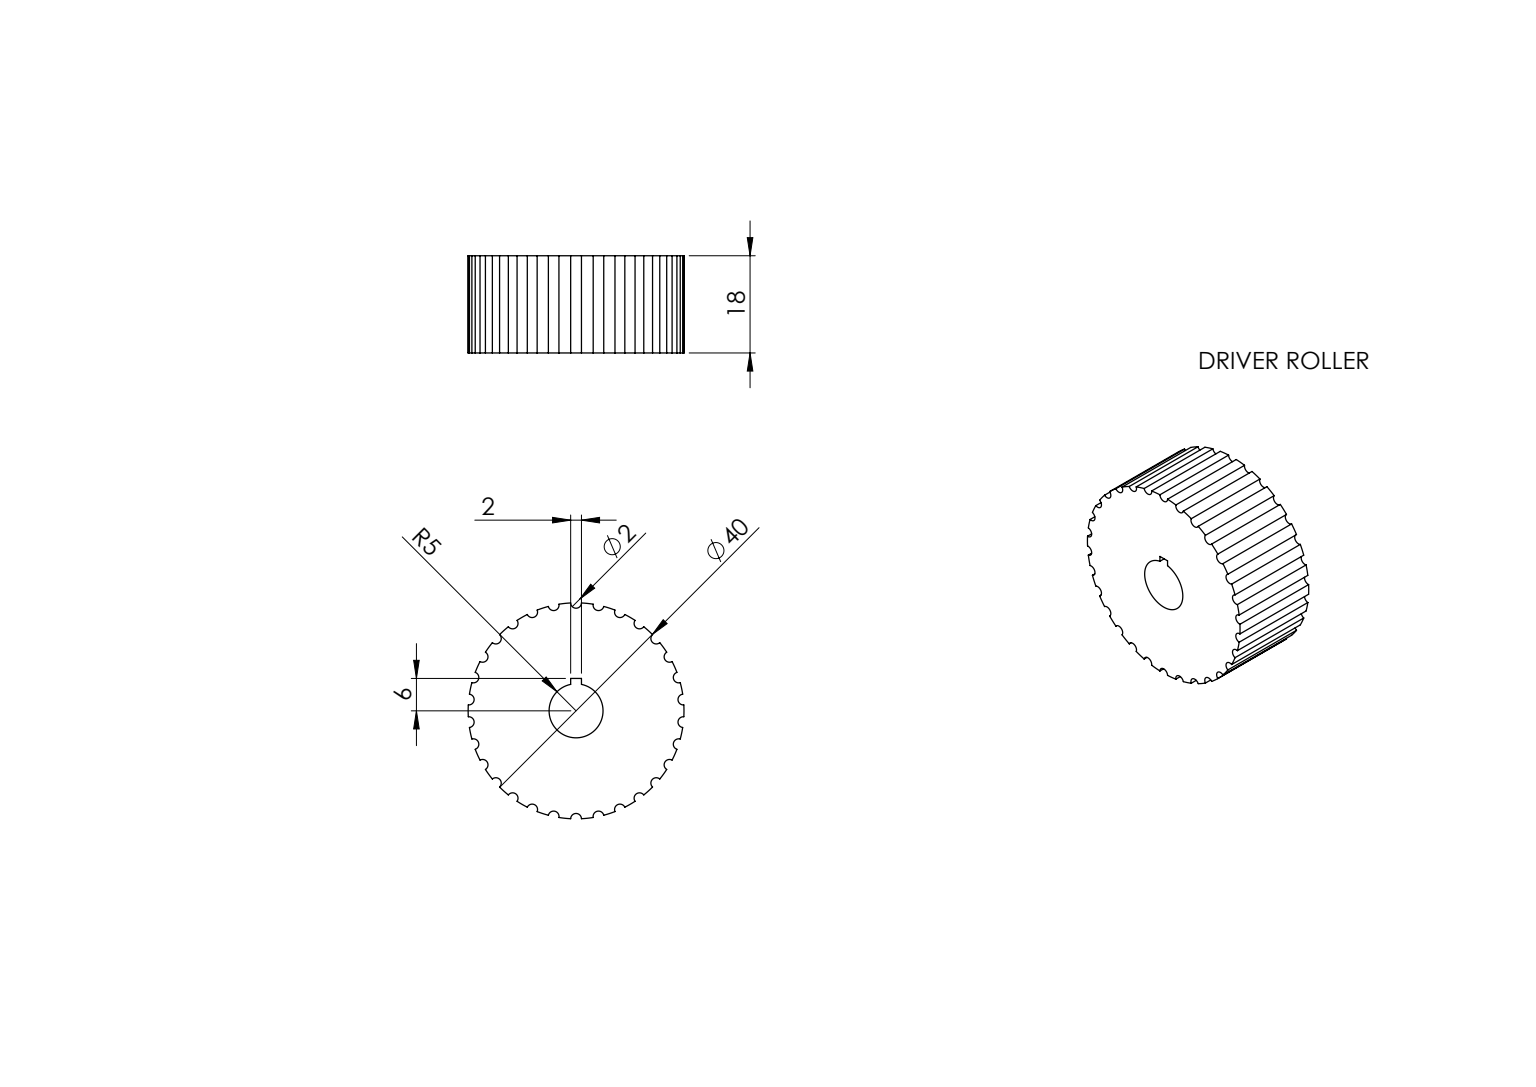
ISO-10303-21;
HEADER;
FILE_DESCRIPTION (('STEP AP214'),
    '1' );
FILE_NAME ('driver roller.step',
    '2026-10-31T03:44:21',
    ( '' ),
    ( '' ),
    'SwSTEP 2.0',
    'SolidWorks 2026',
    '' );
FILE_SCHEMA (( 'AUTOMOTIVE_DESIGN' ));
ENDSEC;

DATA;
#2=ORIENTED_EDGE ( 'NONE', *, *, #6633, .F. ) ;
#14=DIRECTION ( 'NONE',  ( -4.082155997157844188E-16, 1.000000000000000000, 0.000000000000000000 ) ) ;
#47=ORIENTED_EDGE ( 'NONE', *, *, #5852, .F. ) ;
#49=DIRECTION ( 'NONE',  ( -0.000000000000000000, -0.000000000000000000, -1.000000000000000000 ) ) ;
#61=FACE_OUTER_BOUND ( 'NONE', #9370, .T. ) ;
#94=EDGE_LOOP ( 'NONE', ( #13981, #857, #13951, #13577 ) ) ;
#95=DIRECTION ( 'NONE',  ( -1.000000000000000000, 0.000000000000000000, 0.000000000000000000 ) ) ;
#96=ORIENTED_EDGE ( 'NONE', *, *, #2338, .F. ) ;
#114=ORIENTED_EDGE ( 'NONE', *, *, #10804, .F. ) ;
#116=EDGE_CURVE ( 'NONE', #14983, #12413, #19360, .T. ) ;
#117=DIRECTION ( 'NONE',  ( 0.000000000000000000, 0.000000000000000000, 1.000000000000000000 ) ) ;
#121=CARTESIAN_POINT ( 'NONE',  ( -0.9999999999999995559, -15.10102051443364246, 9.000000000000000000 ) ) ;
#129=ORIENTED_EDGE ( 'NONE', *, *, #17684, .F. ) ;
#132=AXIS2_PLACEMENT_3D ( 'NONE', #16115, #16207, #5718 ) ;
#142=DIRECTION ( 'NONE',  ( -0.9781476007338065770, 0.2079116908177552348, 0.000000000000000000 ) ) ;
#145=CIRCLE ( 'NONE', #8274, 20.00000000000000000 ) ;
#152=CARTESIAN_POINT ( 'NONE',  ( 11.75570504584926468, -3.819660112500910198, 9.000000000000000000 ) ) ;
#159=DIRECTION ( 'NONE',  ( 1.000000000000000000, 0.000000000000000000, 0.000000000000000000 ) ) ;
#176=EDGE_CURVE ( 'NONE', #16215, #3087, #11160, .T. ) ;
#177=DIRECTION ( 'NONE',  ( 0.000000000000000000, 0.000000000000000000, 1.000000000000000000 ) ) ;
#179=ORIENTED_EDGE ( 'NONE', *, *, #18456, .F. ) ;
#183=CIRCLE ( 'NONE', #15507, 5.000000000000000888 ) ;
#193=CARTESIAN_POINT ( 'NONE',  ( -3.158233816355059620, -39.56295201467614220, -9.000000000000000000 ) ) ;
#198=CIRCLE ( 'NONE', #9874, 1.000000000000000000 ) ;
#199=CARTESIAN_POINT ( 'NONE',  ( -19.30627432446647163, -14.77814480204146363, 9.000000000000000000 ) ) ;
#209=ORIENTED_EDGE ( 'NONE', *, *, #14535, .T. ) ;
#214=DIRECTION ( 'NONE',  ( -0.000000000000000000, 0.000000000000000000, 1.000000000000000000 ) ) ;
#225=ORIENTED_EDGE ( 'NONE', *, *, #17454, .F. ) ;
#233=DIRECTION ( 'NONE',  ( -0.3090169943749528914, 0.9510565162951518658, 0.000000000000000000 ) ) ;
#250=DIRECTION ( 'NONE',  ( 0.000000000000000000, 0.000000000000000000, 1.000000000000000000 ) ) ;
#256=ORIENTED_EDGE ( 'NONE', *, *, #7357, .T. ) ;
#258=VERTEX_POINT ( 'NONE', #12266 ) ;
#274=DIRECTION ( 'NONE',  ( -0.6691306063588506881, -0.7431448254774009055, 0.000000000000000000 ) ) ;
#277=DIRECTION ( 'NONE',  ( 1.000000000000000000, 0.000000000000000000, 0.000000000000000000 ) ) ;
#279=ORIENTED_EDGE ( 'NONE', *, *, #12618, .T. ) ;
#281=EDGE_CURVE ( 'NONE', #8618, #8760, #1727, .T. ) ;
#300=FACE_OUTER_BOUND ( 'NONE', #17953, .T. ) ;
#309=DIRECTION ( 'NONE',  ( -0.000000000000000000, -0.000000000000000000, -1.000000000000000000 ) ) ;
#310=ORIENTED_EDGE ( 'NONE', *, *, #4548, .T. ) ;
#313=CIRCLE ( 'NONE', #4397, 1.000000000000000444 ) ;
#317=DIRECTION ( 'NONE',  ( 0.000000000000000000, 0.000000000000000000, 1.000000000000000000 ) ) ;
#327=CARTESIAN_POINT ( 'NONE',  ( 0.000000000000000000, 0.000000000000000000, -9.000000000000000000 ) ) ;
#329=ORIENTED_EDGE ( 'NONE', *, *, #6092, .T. ) ;
#337=VERTEX_POINT ( 'NONE', #4121 ) ;
#348=DIRECTION ( 'NONE',  ( -0.000000000000000000, -0.000000000000000000, -1.000000000000000000 ) ) ;
#354=ORIENTED_EDGE ( 'NONE', *, *, #1026, .F. ) ;
#368=FACE_OUTER_BOUND ( 'NONE', #2307, .T. ) ;
#376=DIRECTION ( 'NONE',  ( -0.000000000000000000, -0.000000000000000000, 1.000000000000000000 ) ) ;
#382=AXIS2_PLACEMENT_3D ( 'NONE', #14726, #11588, #19073 ) ;
#383=DIRECTION ( 'NONE',  ( 0.000000000000000000, 0.000000000000000000, 1.000000000000000000 ) ) ;
#388=ORIENTED_EDGE ( 'NONE', *, *, #14666, .F. ) ;
#392=DIRECTION ( 'NONE',  ( 0.000000000000000000, 0.000000000000000000, -1.000000000000000000 ) ) ;
#399=( LENGTH_UNIT ( ) NAMED_UNIT ( * ) SI_UNIT ( .MILLI., .METRE. ) );
#403=DIRECTION ( 'NONE',  ( 0.000000000000000000, 0.000000000000000000, -1.000000000000000000 ) ) ;
#408=DIRECTION ( 'NONE',  ( 0.000000000000000000, 0.000000000000000000, 1.000000000000000000 ) ) ;
#428=ORIENTED_EDGE ( 'NONE', *, *, #9768, .T. ) ;
#437=DIRECTION ( 'NONE',  ( 0.000000000000000000, 0.000000000000000000, 1.000000000000000000 ) ) ;
#438=CIRCLE ( 'NONE', #9207, 1.000000000000000222 ) ;
#439=VERTEX_POINT ( 'NONE', #4586 ) ;
#462=DIRECTION ( 'NONE',  ( 0.000000000000000000, 0.000000000000000000, 1.000000000000000000 ) ) ;
#469=FACE_OUTER_BOUND ( 'NONE', #1033, .T. ) ;
#494=CIRCLE ( 'NONE', #15524, 1.000000000000000666 ) ;
#508=VERTEX_POINT ( 'NONE', #6242 ) ;
#513=DIRECTION ( 'NONE',  ( 0.9781476007338055778, 0.2079116908177597867, 0.000000000000000000 ) ) ;
#520=CARTESIAN_POINT ( 'NONE',  ( -19.97007065299861850, -18.90625500492885180, -9.000000000000000000 ) ) ;
#526=DIRECTION ( 'NONE',  ( -0.000000000000000000, -0.000000000000000000, 1.000000000000000000 ) ) ;
#538=CARTESIAN_POINT ( 'NONE',  ( -14.17539641854921229, -5.891203581560112923, 9.000000000000000000 ) ) ;
#542=CARTESIAN_POINT ( 'NONE',  ( -0.9996874511566050669, -39.97499999999999432, 9.000000000000000000 ) ) ;
#543=ORIENTED_EDGE ( 'NONE', *, *, #13837, .F. ) ;
#550=DIRECTION ( 'NONE',  ( -0.000000000000000000, 0.000000000000000000, -1.000000000000000000 ) ) ;
#555=CARTESIAN_POINT ( 'NONE',  ( -1.000000000000000000, -14.00000000000000000, 8.999999999999998224 ) ) ;
#564=ORIENTED_EDGE ( 'NONE', *, *, #16830, .T. ) ;
#567=CARTESIAN_POINT ( 'NONE',  ( 17.79870116617236420, -10.87825472854593301, 9.000000000000000000 ) ) ;
#571=CARTESIAN_POINT ( 'NONE',  ( 18.68843350152500093, -27.12337372732038432, 0.000000000000000000 ) ) ;
#575=EDGE_CURVE ( 'NONE', #17511, #6795, #14148, .T. ) ;
#583=( NAMED_UNIT ( * ) SI_UNIT ( $, .STERADIAN. ) SOLID_ANGLE_UNIT ( ) );
#585=VERTEX_POINT ( 'NONE', #10450 ) ;
#595=LINE ( 'NONE', #15210, #9936 ) ;
#597=CARTESIAN_POINT ( 'NONE',  ( -10.93224627749309796, -3.252283996668733135, 0.000000000000000000 ) ) ;
#620=CARTESIAN_POINT ( 'NONE',  ( -11.75570504584948139, -3.819660112501066518, -9.000000000000000000 ) ) ;
#625=CIRCLE ( 'NONE', #12841, 20.00000000000000000 ) ;
#630=ORIENTED_EDGE ( 'NONE', *, *, #16372, .F. ) ;
#632=CIRCLE ( 'NONE', #5645, 1.000000000000000000 ) ;
#634=FACE_OUTER_BOUND ( 'NONE', #11741, .T. ) ;
#637=EDGE_LOOP ( 'NONE', ( #3972, #2, #1409, #7912 ) ) ;
#660=VERTEX_POINT ( 'NONE', #9650 ) ;
#661=CARTESIAN_POINT ( 'NONE',  ( -9.037824375505556063, -2.158539001597498341, 9.000000000000000000 ) ) ;
#666=VERTEX_POINT ( 'NONE', #11028 ) ;
#667=ORIENTED_EDGE ( 'NONE', *, *, #12974, .T. ) ;
#668=DIRECTION ( 'NONE',  ( -0.6691306063588624564, 0.7431448254773903583, 0.000000000000000000 ) ) ;
#673=ORIENTED_EDGE ( 'NONE', *, *, #4548, .F. ) ;
#677=CARTESIAN_POINT ( 'NONE',  ( -18.89043790736547379, -17.90943073464699609, -9.000000000000000000 ) ) ;
#681=VECTOR ( 'NONE', #14209, 1000.000000000000000 ) ;
#686=FACE_OUTER_BOUND ( 'NONE', #12366, .T. ) ;
#695=DIRECTION ( 'NONE',  ( 1.000000000000000000, 0.000000000000000000, 0.000000000000000000 ) ) ;
#716=CARTESIAN_POINT ( 'NONE',  ( -4.158233816355060064, -39.56295201467614220, 9.000000000000000000 ) ) ;
#721=CARTESIAN_POINT ( 'NONE',  ( 17.32050807568887052, -29.99999999999984013, 9.000000000000000000 ) ) ;
#727=ORIENTED_EDGE ( 'NONE', *, *, #14442, .F. ) ;
#747=CARTESIAN_POINT ( 'NONE',  ( 2.449293598294706513E-15, -20.00000000000000000, -9.000000000000000000 ) ) ;
#753=CIRCLE ( 'NONE', #14189, 20.00000000000000000 ) ;
#756=ORIENTED_EDGE ( 'NONE', *, *, #9160, .F. ) ;
#761=CARTESIAN_POINT ( 'NONE',  ( 19.76107906696387317, -16.91783288752825243, -9.000000000000000000 ) ) ;
#765=CARTESIAN_POINT ( 'NONE',  ( -4.999999999999998224, -20.00000000000000000, -8.999999999999998224 ) ) ;
#776=DIRECTION ( 'NONE',  ( -1.000000000000000000, 0.000000000000000000, 0.000000000000000000 ) ) ;
#777=SURFACE_STYLE_FILL_AREA ( #6555 ) ;
#783=EDGE_CURVE ( 'NONE', #14027, #16215, #3977, .T. ) ;
#791=CARTESIAN_POINT ( 'NONE',  ( -11.75570504584948139, -3.819660112501066518, -9.000000000000000000 ) ) ;
#811=CARTESIAN_POINT ( 'NONE',  ( 3.175194142251959395, -0.2536549670829222891, 0.000000000000000000 ) ) ;
#826=EDGE_LOOP ( 'NONE', ( #10240, #13120, #5556, #14929, #17534, #17311, #15195, #957, #13396, #3693, #849, #8118, #17435, #10866, #18404, #3444, #17944, #1819, #10052, #1799, #14812, #13494, #6030, #667, #4210, #4378, #19128, #14482, #9173, #14661, #18119, #5853, #10615, #17650, #8610, #6461, #354, #8873, #329, #14105, #1118, #11724, #12303, #13901, #12807, #3007, #1875, #3118, #11250, #3617, #6139, #1702, #5470, #3801, #428, #9248, #2440, #8586, #4995, #5364, #10159, #6076, #14755, #11333, #9586, #2359, #9658, #10533, #5646, #225, #18731, #17801, #14491, #16083, #10253 ) ) ;
#827=CARTESIAN_POINT ( 'NONE',  ( -0.9996874511566102850, -0.02500000000000036915, 0.000000000000000000 ) ) ;
#847=LINE ( 'NONE', #6820, #14709 ) ;
#849=ORIENTED_EDGE ( 'NONE', *, *, #8720, .T. ) ;
#857=ORIENTED_EDGE ( 'NONE', *, *, #18164, .T. ) ;
#858=DIRECTION ( 'NONE',  ( -0.9781476007338035794, -0.2079116908177690293, 0.000000000000000000 ) ) ;
#864=CYLINDRICAL_SURFACE ( 'NONE', #15186, 20.00000000000000000 ) ;
#865=CARTESIAN_POINT ( 'NONE',  ( 2.449293598294706513E-15, -20.00000000000000000, -9.000000000000000000 ) ) ;
#871=FACE_OUTER_BOUND ( 'NONE', #2850, .T. ) ;
#882=CARTESIAN_POINT ( 'NONE',  ( -8.134732861515892921, -38.27090915285207018, -9.000000000000000000 ) ) ;
#887=DIRECTION ( 'NONE',  ( -0.000000000000000000, -0.000000000000000000, 1.000000000000000000 ) ) ;
#892=EDGE_CURVE ( 'NONE', #16569, #17921, #12589, .T. ) ;
#910=CARTESIAN_POINT ( 'NONE',  ( -13.86289650954781649, -33.38261212717723936, 9.000000000000000000 ) ) ;
#911=CIRCLE ( 'NONE', #12183, 20.00000000000000000 ) ;
#914=CARTESIAN_POINT ( 'NONE',  ( 14.86289650954800479, -33.38261212717704041, 9.000000000000000000 ) ) ;
#922=ORIENTED_EDGE ( 'NONE', *, *, #17197, .T. ) ;
#924=ORIENTED_EDGE ( 'NONE', *, *, #9379, .T. ) ;
#925=CIRCLE ( 'NONE', #14378, 5.000000000000000888 ) ;
#930=ADVANCED_FACE ( 'NONE', ( #3195 ), #3277, .F. ) ;
#934=EDGE_CURVE ( 'NONE', #17942, #4148, #5717, .T. ) ;
#956=ORIENTED_EDGE ( 'NONE', *, *, #13692, .F. ) ;
#957=ORIENTED_EDGE ( 'NONE', *, *, #12323, .T. ) ;
#958=CARTESIAN_POINT ( 'NONE',  ( -19.97007065299861850, -18.90625500492883759, 0.000000000000000000 ) ) ;
#959=VECTOR ( 'NONE', #17165, 1000.000000000000000 ) ;
#972=AXIS2_PLACEMENT_3D ( 'NONE', #4310, #13228, #1180 ) ;
#975=ORIENTED_EDGE ( 'NONE', *, *, #9791, .F. ) ;
#978=( NAMED_UNIT ( * ) SI_UNIT ( $, .STERADIAN. ) SOLID_ANGLE_UNIT ( ) );
#1005=DIRECTION ( 'NONE',  ( 1.000000000000000000, 0.000000000000000000, -0.000000000000000000 ) ) ;
#1023=DIRECTION ( 'NONE',  ( 0.000000000000000000, 0.000000000000000000, 1.000000000000000000 ) ) ;
#1026=EDGE_CURVE ( 'NONE', #2792, #1052, #11194, .T. ) ;
#1030=DIRECTION ( 'NONE',  ( 0.000000000000000000, 0.000000000000000000, -1.000000000000000000 ) ) ;
#1033=EDGE_LOOP ( 'NONE', ( #9433, #14051, #16065, #10439 ) ) ;
#1039=ORIENTED_EDGE ( 'NONE', *, *, #14682, .T. ) ;
#1050=ORIENTED_EDGE ( 'NONE', *, *, #3071, .T. ) ;
#1051=LINE ( 'NONE', #19006, #12176 ) ;
#1052=VERTEX_POINT ( 'NONE', #16911 ) ;
#1055=VERTEX_POINT ( 'NONE', #15422 ) ;
#1057=CARTESIAN_POINT ( 'NONE',  ( 2.449293598294706513E-15, -20.00000000000000000, -9.000000000000000000 ) ) ;
#1072=ORIENTED_EDGE ( 'NONE', *, *, #2201, .F. ) ;
#1077=ORIENTED_EDGE ( 'NONE', *, *, #13125, .F. ) ;
#1086=CARTESIAN_POINT ( 'NONE',  ( -19.76107906696389094, -23.08216711247160546, 0.000000000000000000 ) ) ;
#1087=DIRECTION ( 'NONE',  ( 1.000000000000000000, 0.000000000000000000, 0.000000000000000000 ) ) ;
#1101=AXIS2_PLACEMENT_3D ( 'NONE', #11279, #9807, #15805 ) ;
#1105=CARTESIAN_POINT ( 'NONE',  ( -15.51323935927274711, -7.377028694403568565, -9.000000000000000000 ) ) ;
#1113=DIRECTION ( 'NONE',  ( -0.000000000000000000, -0.000000000000000000, 1.000000000000000000 ) ) ;
#1114=CIRCLE ( 'NONE', #14881, 0.9999999999999995559 ) ;
#1115=ORIENTED_EDGE ( 'NONE', *, *, #14633, .F. ) ;
#1118=ORIENTED_EDGE ( 'NONE', *, *, #14777, .T. ) ;
#1129=AXIS2_PLACEMENT_3D ( 'NONE', #6537, #12520, #3514 ) ;
#1133=EDGE_CURVE ( 'NONE', #17716, #14101, #19058, .T. ) ;
#1139=FACE_OUTER_BOUND ( 'NONE', #2590, .T. ) ;
#1144=FACE_OUTER_BOUND ( 'NONE', #5875, .T. ) ;
#1150=CARTESIAN_POINT ( 'NONE',  ( -9.037824375505429941, -37.84146099840256738, -9.000000000000000000 ) ) ;
#1153=DIRECTION ( 'NONE',  ( 0.000000000000000000, -0.000000000000000000, -1.000000000000000000 ) ) ;
#1154=ORIENTED_EDGE ( 'NONE', *, *, #10481, .T. ) ;
#1159=VECTOR ( 'NONE', #3094, 1000.000000000000000 ) ;
#1166=ORIENTED_EDGE ( 'NONE', *, *, #17313, .T. ) ;
#1170=DIRECTION ( 'NONE',  ( 0.000000000000000000, 0.000000000000000000, -1.000000000000000000 ) ) ;
#1180=DIRECTION ( 'NONE',  ( 1.000000000000000000, 0.000000000000000000, 0.000000000000000000 ) ) ;
#1182=AXIS2_PLACEMENT_3D ( 'NONE', #7159, #887, #17373 ) ;
#1185=VECTOR ( 'NONE', #1170, 1000.000000000000000 ) ;
#1196=DIRECTION ( 'NONE',  ( 0.9135454576426006446, 0.4067366430758008189, 0.000000000000000000 ) ) ;
#1201=CARTESIAN_POINT ( 'NONE',  ( 19.97007065299861139, -18.90625500492856759, 9.000000000000000000 ) ) ;
#1216=ORIENTED_EDGE ( 'NONE', *, *, #14103, .F. ) ;
#1220=VECTOR ( 'NONE', #3702, 1000.000000000000000 ) ;
#1234=CYLINDRICAL_SURFACE ( 'NONE', #12250, 20.00000000000000000 ) ;
#1236=VECTOR ( 'NONE', #3578, 1000.000000000000000 ) ;
#1248=CARTESIAN_POINT ( 'NONE',  ( 19.02113032590313679, -26.18033988749876428, -9.000000000000000000 ) ) ;
#1249=DIRECTION ( 'NONE',  ( 1.000000000000000000, 0.000000000000000000, 0.000000000000000000 ) ) ;
#1251=VERTEX_POINT ( 'NONE', #9338 ) ;
#1254=VECTOR ( 'NONE', #13053, 1000.000000000000000 ) ;
#1255=CYLINDRICAL_SURFACE ( 'NONE', #14463, 1.000000000000000888 ) ;
#1269=CIRCLE ( 'NONE', #13151, 1.000000000000001554 ) ;
#1275=AXIS2_PLACEMENT_3D ( 'NONE', #4500, #177, #5766 ) ;
#1278=AXIS2_PLACEMENT_3D ( 'NONE', #9226, #5014, #3552 ) ;
#1279=ORIENTED_EDGE ( 'NONE', *, *, #7480, .T. ) ;
#1280=ORIENTED_EDGE ( 'NONE', *, *, #2081, .T. ) ;
#1288=CIRCLE ( 'NONE', #12233, 0.9999999999999995559 ) ;
#1290=AXIS2_PLACEMENT_3D ( 'NONE', #10129, #14632, #19085 ) ;
#1316=ORIENTED_EDGE ( 'NONE', *, *, #6301, .F. ) ;
#1323=EDGE_LOOP ( 'NONE', ( #6367, #5280, #1972, #14556 ) ) ;
#1331=CARTESIAN_POINT ( 'NONE',  ( -9.037824375505556063, -2.158539001597497897, 0.000000000000000000 ) ) ;
#1354=ADVANCED_FACE ( 'NONE', ( #14435 ), #4150, .F. ) ;
#1355=DIRECTION ( 'NONE',  ( 0.3090169943749560000, -0.9510565162951507556, 0.000000000000000000 ) ) ;
#1358=ORIENTED_EDGE ( 'NONE', *, *, #5669, .T. ) ;
#1360=ORIENTED_EDGE ( 'NONE', *, *, #9091, .F. ) ;
#1365=CARTESIAN_POINT ( 'NONE',  ( 14.17539641854901689, -5.891203581559917524, 9.000000000000000000 ) ) ;
#1374=DIRECTION ( 'NONE',  ( -1.000000000000000000, 0.000000000000000000, 0.000000000000000000 ) ) ;
#1408=ORIENTED_EDGE ( 'NONE', *, *, #9197, .F. ) ;
#1409=ORIENTED_EDGE ( 'NONE', *, *, #16613, .T. ) ;
#1412=AXIS2_PLACEMENT_3D ( 'NONE', #1715, #16627, #18202 ) ;
#1429=AXIS2_PLACEMENT_3D ( 'NONE', #18167, #4723, #9307 ) ;
#1435=CYLINDRICAL_SURFACE ( 'NONE', #15616, 20.00000000000000000 ) ;
#1438=DIRECTION ( 'NONE',  ( 0.000000000000000000, 0.000000000000000000, 1.000000000000000000 ) ) ;
#1441=CIRCLE ( 'NONE', #8001, 0.9999999999999980016 ) ;
#1443=ORIENTED_EDGE ( 'NONE', *, *, #14434, .F. ) ;
#1447=DIRECTION ( 'NONE',  ( 1.000000000000000000, 0.000000000000000000, 0.000000000000000000 ) ) ;
#1456=ORIENTED_EDGE ( 'NONE', *, *, #2108, .T. ) ;
#1461=DIRECTION ( 'NONE',  ( 0.000000000000000000, 0.000000000000000000, 1.000000000000000000 ) ) ;
#1482=AXIS2_PLACEMENT_3D ( 'NONE', #7732, #10568, #12243 ) ;
#1492=AXIS2_PLACEMENT_3D ( 'NONE', #15841, #9755, #5350 ) ;
#1493=CARTESIAN_POINT ( 'NONE',  ( -19.89043790736547379, -17.90943073464699609, -9.000000000000000000 ) ) ;
#1496=CARTESIAN_POINT ( 'NONE',  ( -17.32050807568879236, -10.00000000000004263, -9.000000000000000000 ) ) ;
#1513=FACE_OUTER_BOUND ( 'NONE', #15002, .T. ) ;
#1523=CYLINDRICAL_SURFACE ( 'NONE', #1412, 20.00000000000000000 ) ;
#1526=CARTESIAN_POINT ( 'NONE',  ( 19.89043790736549155, -22.09056926535286891, 9.000000000000000000 ) ) ;
#1529=ORIENTED_EDGE ( 'NONE', *, *, #13719, .F. ) ;
#1531=EDGE_LOOP ( 'NONE', ( #1965, #8200, #6115, #16241 ) ) ;
#1533=AXIS2_PLACEMENT_3D ( 'NONE', #1751, #10657, #4699 ) ;
#1542=CYLINDRICAL_SURFACE ( 'NONE', #4122, 20.00000000000000000 ) ;
#1556=EDGE_CURVE ( 'NONE', #12796, #4767, #6808, .T. ) ;
#1578=CARTESIAN_POINT ( 'NONE',  ( -0.9999999999999976685, -20.00000000000000000, 8.999999999999998224 ) ) ;
#1581=LINE ( 'NONE', #10578, #15025 ) ;
#1585=FACE_OUTER_BOUND ( 'NONE', #1531, .T. ) ;
#1591=CARTESIAN_POINT ( 'NONE',  ( 2.449293598294706513E-15, -20.00000000000000000, 9.000000000000000000 ) ) ;
#1600=CARTESIAN_POINT ( 'NONE',  ( -18.89043790736547379, -17.90943073464699609, 9.000000000000000000 ) ) ;
#1603=ADVANCED_FACE ( 'NONE', ( #8937 ), #14920, .F. ) ;
#1608=ORIENTED_EDGE ( 'NONE', *, *, #6329, .F. ) ;
#1610=CIRCLE ( 'NONE', #3790, 0.9999999999999993339 ) ;
#1611=ORIENTED_EDGE ( 'NONE', *, *, #14954, .T. ) ;
#1612=CIRCLE ( 'NONE', #10047, 0.9999999999999997780 ) ;
#1633=EDGE_CURVE ( 'NONE', #2794, #3573, #8136, .T. ) ;
#1635=DIRECTION ( 'NONE',  ( -0.000000000000000000, -0.000000000000000000, -1.000000000000000000 ) ) ;
#1643=VERTEX_POINT ( 'NONE', #4823 ) ;
#1646=CIRCLE ( 'NONE', #5709, 20.00000000000000000 ) ;
#1651=LINE ( 'NONE', #6240, #4142 ) ;
#1677=EDGE_CURVE ( 'NONE', #12007, #15146, #3992, .T. ) ;
#1702=ORIENTED_EDGE ( 'NONE', *, *, #16732, .F. ) ;
#1703=VECTOR ( 'NONE', #3262, 1000.000000000000000 ) ;
#1709=CYLINDRICAL_SURFACE ( 'NONE', #10850, 20.00000000000000000 ) ;
#1715=CARTESIAN_POINT ( 'NONE',  ( 2.449293598294706513E-15, -20.00000000000000000, 9.000000000000000000 ) ) ;
#1727=CIRCLE ( 'NONE', #3925, 20.00000000000000000 ) ;
#1730=CARTESIAN_POINT ( 'NONE',  ( 2.449293598294706513E-15, -20.00000000000000000, 9.000000000000000000 ) ) ;
#1733=EDGE_CURVE ( 'NONE', #4148, #11140, #595, .T. ) ;
#1736=DIRECTION ( 'NONE',  ( -1.000000000000000000, 0.000000000000000000, 0.000000000000000000 ) ) ;
#1751=CARTESIAN_POINT ( 'NONE',  ( -8.134732861515892921, -38.27090915285207018, -9.000000000000000000 ) ) ;
#1752=CIRCLE ( 'NONE', #7684, 0.9999999999999985567 ) ;
#1754=CARTESIAN_POINT ( 'NONE',  ( 17.32050807568887052, -29.99999999999984013, -9.000000000000000000 ) ) ;
#1758=EDGE_CURVE ( 'NONE', #3235, #16171, #4029, .T. ) ;
#1761=VERTEX_POINT ( 'NONE', #4126 ) ;
#1766=VECTOR ( 'NONE', #7150, 1000.000000000000000 ) ;
#1771=PLANE ( 'NONE',  #2184 ) ;
#1772=AXIS2_PLACEMENT_3D ( 'NONE', #9114, #19244, #8723 ) ;
#1774=CARTESIAN_POINT ( 'NONE',  ( -14.86289650954790886, -6.617387872822862782, -9.000000000000000000 ) ) ;
#1777=ORIENTED_EDGE ( 'NONE', *, *, #4947, .T. ) ;
#1790=CARTESIAN_POINT ( 'NONE',  ( 2.449293598294706513E-15, -20.00000000000000000, -9.000000000000000000 ) ) ;
#1797=ADVANCED_FACE ( 'NONE', ( #8328 ), #14308, .F. ) ;
#1798=AXIS2_PLACEMENT_3D ( 'NONE', #18363, #8031, #10881 ) ;
#1799=ORIENTED_EDGE ( 'NONE', *, *, #4544, .F. ) ;
#1807=LINE ( 'NONE', #16713, #1159 ) ;
#1816=VECTOR ( 'NONE', #550, 1000.000000000000000 ) ;
#1819=ORIENTED_EDGE ( 'NONE', *, *, #10875, .T. ) ;
#1829=DIRECTION ( 'NONE',  ( -0.000000000000000000, -0.000000000000000000, 1.000000000000000000 ) ) ;
#1834=DIRECTION ( 'NONE',  ( 0.000000000000000000, 0.000000000000000000, 1.000000000000000000 ) ) ;
#1841=EDGE_CURVE ( 'NONE', #16171, #2874, #10835, .T. ) ;
#1844=ORIENTED_EDGE ( 'NONE', *, *, #13469, .F. ) ;
#1852=DIRECTION ( 'NONE',  ( 0.000000000000000000, 0.000000000000000000, 1.000000000000000000 ) ) ;
#1857=VERTEX_POINT ( 'NONE', #199 ) ;
#1858=CIRCLE ( 'NONE', #4353, 0.9999999999999995559 ) ;
#1860=EDGE_CURVE ( 'NONE', #16340, #14634, #12716, .T. ) ;
#1871=EDGE_CURVE ( 'NONE', #8171, #3999, #4270, .T. ) ;
#1873=DIRECTION ( 'NONE',  ( -0.000000000000000000, -0.000000000000000000, -1.000000000000000000 ) ) ;
#1875=ORIENTED_EDGE ( 'NONE', *, *, #10485, .T. ) ;
#1880=CARTESIAN_POINT ( 'NONE',  ( -16.32050807568879236, -10.00000000000004263, -9.000000000000000000 ) ) ;
#1881=CARTESIAN_POINT ( 'NONE',  ( 8.134732861515777458, -1.729090847147875198, 9.000000000000000000 ) ) ;
#1904=CYLINDRICAL_SURFACE ( 'NONE', #12420, 1.000000000000000888 ) ;
#1913=CIRCLE ( 'NONE', #15365, 0.9999999999999980016 ) ;
#1928=DIRECTION ( 'NONE',  ( 1.000000000000000000, 0.000000000000000000, 0.000000000000000000 ) ) ;
#1940=STYLED_ITEM('',(#19454),#2528);
#1946=ORIENTED_EDGE ( 'NONE', *, *, #5411, .T. ) ;
#1962=DIRECTION ( 'NONE',  ( -0.1045284632676563297, 0.9945218953682731788, 0.000000000000000000 ) ) ;
#1965=ORIENTED_EDGE ( 'NONE', *, *, #19295, .F. ) ;
#1968=ORIENTED_EDGE ( 'NONE', *, *, #15149, .F. ) ;
#1971=AXIS2_PLACEMENT_3D ( 'NONE', #5961, #1834, #12217 ) ;
#1972=ORIENTED_EDGE ( 'NONE', *, *, #14831, .T. ) ;
#1973=CARTESIAN_POINT ( 'NONE',  ( -17.32050807568872841, -30.00000000000008171, 9.000000000000000000 ) ) ;
#1977=DIRECTION ( 'NONE',  ( -0.8090169943749487835, 0.5877852522924713607, 0.000000000000000000 ) ) ;
#1987=EDGE_CURVE ( 'NONE', #15553, #8337, #8329, .T. ) ;
#1991=EDGE_CURVE ( 'NONE', #5469, #3727, #10197, .T. ) ;
#1998=DIRECTION ( 'NONE',  ( 0.9135454576426060846, -0.4067366430757887730, 0.000000000000000000 ) ) ;
#2005=DIRECTION ( 'NONE',  ( -0.000000000000000000, -0.000000000000000000, 1.000000000000000000 ) ) ;
#2009=CYLINDRICAL_SURFACE ( 'NONE', #10982, 1.000000000000000000 ) ;
#2034=DIRECTION ( 'NONE',  ( -0.8090169943749487835, 0.5877852522924713607, 0.000000000000000000 ) ) ;
#2039=LINE ( 'NONE', #18425, #5584 ) ;
#2046=AXIS2_PLACEMENT_3D ( 'NONE', #16246, #19409, #10633 ) ;
#2051=DIRECTION ( 'NONE',  ( 0.000000000000000000, -0.000000000000000000, 1.000000000000000000 ) ) ;
#2055=CARTESIAN_POINT ( 'NONE',  ( 2.449293598294706513E-15, -20.00000000000000000, 9.000000000000000000 ) ) ;
#2058=ORIENTED_EDGE ( 'NONE', *, *, #12323, .F. ) ;
#2060=DIRECTION ( 'NONE',  ( 0.6691306063588571273, 0.7431448254773952433, 0.000000000000000000 ) ) ;
#2067=AXIS2_PLACEMENT_3D ( 'NONE', #11136, #18334, #7818 ) ;
#2069=UNCERTAINTY_MEASURE_WITH_UNIT (LENGTH_MEASURE( 1.000000000000000082E-05 ), #15917, 'distance_accuracy_value', 'NONE');
#2081=EDGE_CURVE ( 'NONE', #8420, #10947, #6442, .T. ) ;
#2099=DIRECTION ( 'NONE',  ( 1.000000000000000000, 0.000000000000000000, 0.000000000000000000 ) ) ;
#2108=EDGE_CURVE ( 'NONE', #14634, #8760, #16789, .T. ) ;
#2110=LINE ( 'NONE', #14243, #4354 ) ;
#2120=CARTESIAN_POINT ( 'NONE',  ( -11.75570504584937481, -36.18033988749900942, -9.000000000000000000 ) ) ;
#2151=VECTOR ( 'NONE', #2567, 1000.000000000000000 ) ;
#2160=LINE ( 'NONE', #6554, #4949 ) ;
#2161=CARTESIAN_POINT ( 'NONE',  ( 8.134732861516145164, -38.27090915285195649, 9.000000000000000000 ) ) ;
#2162=ORIENTED_EDGE ( 'NONE', *, *, #1991, .T. ) ;
#2176=CARTESIAN_POINT ( 'NONE',  ( 2.449293598294706513E-15, -20.00000000000000000, 9.000000000000000000 ) ) ;
#2180=AXIS2_PLACEMENT_3D ( 'NONE', #152, #15340, #15435 ) ;
#2184=AXIS2_PLACEMENT_3D ( 'NONE', #13721, #6272, #18520 ) ;
#2198=CIRCLE ( 'NONE', #5319, 20.00000000000000000 ) ;
#2199=CARTESIAN_POINT ( 'NONE',  ( 2.449293598294706513E-15, -20.00000000000000000, -9.000000000000000000 ) ) ;
#2201=EDGE_CURVE ( 'NONE', #439, #4800, #15844, .T. ) ;
#2219=CARTESIAN_POINT ( 'NONE',  ( 2.449293598294706513E-15, -20.00000000000000000, 9.000000000000000000 ) ) ;
#2221=EDGE_LOOP ( 'NONE', ( #8383, #13069, #10157, #7169 ) ) ;
#2247=EDGE_CURVE ( 'NONE', #6336, #11140, #18043, .T. ) ;
#2250=ORIENTED_EDGE ( 'NONE', *, *, #3903, .F. ) ;
#2266=ORIENTED_EDGE ( 'NONE', *, *, #8508, .F. ) ;
#2269=ORIENTED_EDGE ( 'NONE', *, *, #3289, .T. ) ;
#2298=CARTESIAN_POINT ( 'NONE',  ( -1.000000000000000000, -14.00000000000000000, -9.000000000000001776 ) ) ;
#2299=DIRECTION ( 'NONE',  ( 0.3090169943749456194, 0.9510565162951541973, 0.000000000000000000 ) ) ;
#2305=DIRECTION ( 'NONE',  ( 0.000000000000000000, -0.000000000000000000, 1.000000000000000000 ) ) ;
#2307=EDGE_LOOP ( 'NONE', ( #16494, #1050, #12634, #12539 ) ) ;
#2308=EDGE_LOOP ( 'NONE', ( #16052, #1529, #4400, #11353 ) ) ;
#2310=DIRECTION ( 'NONE',  ( 0.000000000000000000, 0.000000000000000000, 1.000000000000000000 ) ) ;
#2312=EDGE_CURVE ( 'NONE', #258, #18021, #11756, .T. ) ;
#2319=EDGE_LOOP ( 'NONE', ( #2337, #1408, #3345, #11618 ) ) ;
#2323=CIRCLE ( 'NONE', #2951, 20.00000000000000000 ) ;
#2325=CARTESIAN_POINT ( 'NONE',  ( -3.175194142252219631, -0.2536549670829674197, 9.000000000000000000 ) ) ;
#2337=ORIENTED_EDGE ( 'NONE', *, *, #7587, .F. ) ;
#2338=EDGE_CURVE ( 'NONE', #15553, #16440, #4198, .T. ) ;
#2343=ORIENTED_EDGE ( 'NONE', *, *, #1860, .F. ) ;
#2346=CYLINDRICAL_SURFACE ( 'NONE', #15218, 20.00000000000000000 ) ;
#2349=DIRECTION ( 'NONE',  ( 0.000000000000000000, 0.000000000000000000, 1.000000000000000000 ) ) ;
#2351=EDGE_CURVE ( 'NONE', #1251, #11082, #4294, .T. ) ;
#2359=ORIENTED_EDGE ( 'NONE', *, *, #16613, .F. ) ;
#2364=CARTESIAN_POINT ( 'NONE',  ( -13.86289650954781649, -33.38261212717723936, -9.000000000000000000 ) ) ;
#2367=CARTESIAN_POINT ( 'NONE',  ( -11.75570504584948139, -3.819660112501066518, -9.000000000000000000 ) ) ;
#2374=VECTOR ( 'NONE', #11863, 1000.000000000000000 ) ;
#2382=EDGE_CURVE ( 'NONE', #15146, #12413, #6246, .T. ) ;
#2386=LINE ( 'NONE', #8338, #14550 ) ;
#2409=EDGE_CURVE ( 'NONE', #17731, #2854, #7621, .T. ) ;
#2440=ORIENTED_EDGE ( 'NONE', *, *, #14664, .T. ) ;
#2441=ORIENTED_EDGE ( 'NONE', *, *, #8697, .T. ) ;
#2445=ORIENTED_EDGE ( 'NONE', *, *, #14107, .F. ) ;
#2447=DIRECTION ( 'NONE',  ( 1.000000000000000000, 0.000000000000000000, 0.000000000000000000 ) ) ;
#2452=DIRECTION ( 'NONE',  ( 0.000000000000000000, 0.000000000000000000, 1.000000000000000000 ) ) ;
#2463=LINE ( 'NONE', #2364, #7777 ) ;
#2466=EDGE_CURVE ( 'NONE', #3507, #585, #4127, .T. ) ;
#2468=EDGE_LOOP ( 'NONE', ( #5928, #10210, #6351, #4158 ) ) ;
#2469=VECTOR ( 'NONE', #4014, 1000.000000000000000 ) ;
#2471=LINE ( 'NONE', #17464, #9096 ) ;
#2479=CARTESIAN_POINT ( 'NONE',  ( -3.175194142252219631, -0.2536549670829674197, -9.000000000000000000 ) ) ;
#2483=CARTESIAN_POINT ( 'NONE',  ( 2.449293598294706513E-15, -20.00000000000000000, -9.000000000000000000 ) ) ;
#2488=DIRECTION ( 'NONE',  ( 1.000000000000000000, 0.000000000000000000, 0.000000000000000000 ) ) ;
#2507=DIRECTION ( 'NONE',  ( 1.000000000000000000, 0.000000000000000000, 0.000000000000000000 ) ) ;
#2517=CARTESIAN_POINT ( 'NONE',  ( -1.000000000000000000, -14.00000000000000000, -9.000000000000001776 ) ) ;
#2528=MANIFOLD_SOLID_BREP ( 'Cavity1', #9591 ) ;
#2532=CIRCLE ( 'NONE', #2845, 1.000000000000000000 ) ;
#2539=DIRECTION ( 'NONE',  ( -0.000000000000000000, -0.000000000000000000, 1.000000000000000000 ) ) ;
#2545=CARTESIAN_POINT ( 'NONE',  ( 2.449293598294706513E-15, -20.00000000000000000, 9.000000000000000000 ) ) ;
#2547=ORIENTED_EDGE ( 'NONE', *, *, #17206, .F. ) ;
#2549=CARTESIAN_POINT ( 'NONE',  ( 0.9996874511566102850, -0.02500000000000036915, 9.000000000000000000 ) ) ;
#2551=ORIENTED_EDGE ( 'NONE', *, *, #9097, .T. ) ;
#2560=CIRCLE ( 'NONE', #6291, 20.00000000000000000 ) ;
#2562=ORIENTED_EDGE ( 'NONE', *, *, #10149, .F. ) ;
#2563=CYLINDRICAL_SURFACE ( 'NONE', #3714, 20.00000000000000000 ) ;
#2567=DIRECTION ( 'NONE',  ( -0.000000000000000000, -0.000000000000000000, 1.000000000000000000 ) ) ;
#2578=DIRECTION ( 'NONE',  ( -0.000000000000000000, 0.000000000000000000, -1.000000000000000000 ) ) ;
#2580=VECTOR ( 'NONE', #7710, 1000.000000000000000 ) ;
#2585=CARTESIAN_POINT ( 'NONE',  ( 9.037824375505676855, -37.84146099840244659, 0.000000000000000000 ) ) ;
#2590=EDGE_LOOP ( 'NONE', ( #2562, #12083, #16218, #3655 ) ) ;
#2591=DIRECTION ( 'NONE',  ( -9.858538378746663627E-23, 5.031452844637890958E-23, -1.000000000000000000 ) ) ;
#2599=EDGE_LOOP ( 'NONE', ( #3905, #17610, #16646, #4861 ) ) ;
#2609=EDGE_CURVE ( 'NONE', #16569, #8295, #8825, .T. ) ;
#2612=ORIENTED_EDGE ( 'NONE', *, *, #1987, .T. ) ;
#2613=DIRECTION ( 'NONE',  ( 0.000000000000000000, 0.000000000000000000, 1.000000000000000000 ) ) ;
#2615=CARTESIAN_POINT ( 'NONE',  ( -17.79870116617248499, -10.87825472854618170, 9.000000000000000000 ) ) ;
#2617=DIRECTION ( 'NONE',  ( 1.000000000000000000, 0.000000000000000000, 0.000000000000000000 ) ) ;
#2619=DIRECTION ( 'NONE',  ( 0.000000000000000000, -0.000000000000000000, 1.000000000000000000 ) ) ;
#2631=DIRECTION ( 'NONE',  ( 0.000000000000000000, 0.000000000000000000, 1.000000000000000000 ) ) ;
#2632=ORIENTED_EDGE ( 'NONE', *, *, #9379, .F. ) ;
#2635=DIRECTION ( 'NONE',  ( -0.000000000000000000, -0.000000000000000000, -1.000000000000000000 ) ) ;
#2638=EDGE_CURVE ( 'NONE', #3507, #5600, #5380, .T. ) ;
#2648=FACE_OUTER_BOUND ( 'NONE', #9276, .T. ) ;
#2654=LINE ( 'NONE', #15870, #13783 ) ;
#2656=VECTOR ( 'NONE', #7004, 1000.000000000000000 ) ;
#2657=VERTEX_POINT ( 'NONE', #4542 ) ;
#2660=CIRCLE ( 'NONE', #16725, 1.000000000000002665 ) ;
#2671=DIRECTION ( 'NONE',  ( -1.000000000000000000, 0.000000000000000000, 0.000000000000000000 ) ) ;
#2679=DIRECTION ( 'NONE',  ( 1.000000000000000000, 0.000000000000000000, 0.000000000000000000 ) ) ;
#2686=AXIS2_PLACEMENT_3D ( 'NONE', #18484, #5033, #3563 ) ;
#2699=AXIS2_PLACEMENT_3D ( 'NONE', #6753, #12737, #17071 ) ;
#2700=VERTEX_POINT ( 'NONE', #6200 ) ;
#2703=DIRECTION ( 'NONE',  ( -0.000000000000000000, -0.000000000000000000, -1.000000000000000000 ) ) ;
#2724=CARTESIAN_POINT ( 'NONE',  ( -12.54977455159113475, -35.57251292194792569, 9.000000000000000000 ) ) ;
#2728=LINE ( 'NONE', #5842, #16587 ) ;
#2729=ORIENTED_EDGE ( 'NONE', *, *, #9965, .T. ) ;
#2734=DIRECTION ( 'NONE',  ( 0.000000000000000000, 0.000000000000000000, -1.000000000000000000 ) ) ;
#2747=AXIS2_PLACEMENT_3D ( 'NONE', #10199, #16201, #14918 ) ;
#2750=EDGE_LOOP ( 'NONE', ( #14452, #279, #17212, #18930 ) ) ;
#2755=VECTOR ( 'NONE', #6736, 1000.000000000000000 ) ;
#2766=CYLINDRICAL_SURFACE ( 'NONE', #8184, 1.000000000000000000 ) ;
#2779=DIRECTION ( 'NONE',  ( -0.000000000000000000, -0.000000000000000000, 1.000000000000000000 ) ) ;
#2787=CIRCLE ( 'NONE', #9951, 20.00000000000000000 ) ;
#2792=VERTEX_POINT ( 'NONE', #11826 ) ;
#2793=CYLINDRICAL_SURFACE ( 'NONE', #8418, 20.00000000000000000 ) ;
#2794=VERTEX_POINT ( 'NONE', #4100 ) ;
#2798=AXIS2_PLACEMENT_3D ( 'NONE', #1754, #5071, #277 ) ;
#2801=DIRECTION ( 'NONE',  ( -4.082155997157844188E-16, 1.000000000000000000, 0.000000000000000000 ) ) ;
#2811=FACE_OUTER_BOUND ( 'NONE', #15172, .T. ) ;
#2817=ORIENTED_EDGE ( 'NONE', *, *, #176, .F. ) ;
#2823=ORIENTED_EDGE ( 'NONE', *, *, #17798, .F. ) ;
#2824=CYLINDRICAL_SURFACE ( 'NONE', #11268, 20.00000000000000000 ) ;
#2827=ADVANCED_FACE ( 'NONE', ( #2648 ), #1255, .F. ) ;
#2836=CARTESIAN_POINT ( 'NONE',  ( -19.89043790736545603, -22.09056926535314602, -9.000000000000000000 ) ) ;
#2839=EDGE_CURVE ( 'NONE', #4192, #18235, #11010, .T. ) ;
#2842=VERTEX_POINT ( 'NONE', #4287 ) ;
#2845=AXIS2_PLACEMENT_3D ( 'NONE', #1881, #16783, #9309 ) ;
#2848=CIRCLE ( 'NONE', #9701, 20.00000000000000000 ) ;
#2850=EDGE_LOOP ( 'NONE', ( #3388, #18980, #16443, #4274 ) ) ;
#2854=VERTEX_POINT ( 'NONE', #14768 ) ;
#2855=CARTESIAN_POINT ( 'NONE',  ( 2.449293598294706513E-15, -20.00000000000000000, 9.000000000000000000 ) ) ;
#2860=CYLINDRICAL_SURFACE ( 'NONE', #8608, 20.00000000000000000 ) ;
#2863=VECTOR ( 'NONE', #9367, 1000.000000000000000 ) ;
#2869=EDGE_LOOP ( 'NONE', ( #12972, #17232, #17630, #3143 ) ) ;
#2871=CARTESIAN_POINT ( 'NONE',  ( 0.000000000000000000, 0.000000000000000000, 0.000000000000000000 ) ) ;
#2874=VERTEX_POINT ( 'NONE', #6338 ) ;
#2875=CARTESIAN_POINT ( 'NONE',  ( 2.449293598294706513E-15, -20.00000000000000000, 9.000000000000000000 ) ) ;
#2877=DIRECTION ( 'NONE',  ( 0.000000000000000000, 0.000000000000000000, 1.000000000000000000 ) ) ;
#2881=DIRECTION ( 'NONE',  ( -1.000000000000000000, 0.000000000000000000, 0.000000000000000000 ) ) ;
#2883=DIRECTION ( 'NONE',  ( 1.000000000000000000, 0.000000000000000000, 0.000000000000000000 ) ) ;
#2886=FACE_OUTER_BOUND ( 'NONE', #3109, .T. ) ;
#2898=DIRECTION ( 'NONE',  ( 0.000000000000000000, 0.000000000000000000, 1.000000000000000000 ) ) ;
#2900=DIRECTION ( 'NONE',  ( -1.000000000000000000, 0.000000000000000000, 0.000000000000000000 ) ) ;
#2903=CARTESIAN_POINT ( 'NONE',  ( -10.93224627749309796, -3.252283996668732691, 9.000000000000000000 ) ) ;
#2912=ORIENTED_EDGE ( 'NONE', *, *, #4144, .F. ) ;
#2920=DIRECTION ( 'NONE',  ( -0.000000000000000000, -0.000000000000000000, -1.000000000000000000 ) ) ;
#2923=FACE_OUTER_BOUND ( 'NONE', #2750, .T. ) ;
#2924=ORIENTED_EDGE ( 'NONE', *, *, #15484, .T. ) ;
#2928=EDGE_CURVE ( 'NONE', #16215, #2657, #1646, .T. ) ;
#2938=EDGE_CURVE ( 'NONE', #13867, #585, #1651, .T. ) ;
#2951=AXIS2_PLACEMENT_3D ( 'NONE', #4359, #12092, #19393 ) ;
#2984=ORIENTED_EDGE ( 'NONE', *, *, #12318, .T. ) ;
#2998=DIRECTION ( 'NONE',  ( 1.000000000000000000, 0.000000000000000000, 0.000000000000000000 ) ) ;
#3001=CIRCLE ( 'NONE', #4565, 0.9999999999999995559 ) ;
#3002=ADVANCED_FACE ( 'NONE', ( #368 ), #4778, .F. ) ;
#3004=CARTESIAN_POINT ( 'NONE',  ( -8.134732861515892921, -38.27090915285207018, 9.000000000000000000 ) ) ;
#3007=ORIENTED_EDGE ( 'NONE', *, *, #4947, .F. ) ;
#3008=LINE ( 'NONE', #17631, #16571 ) ;
#3016=ORIENTED_EDGE ( 'NONE', *, *, #6565, .F. ) ;
#3017=DIRECTION ( 'NONE',  ( -0.000000000000000000, -0.000000000000000000, -1.000000000000000000 ) ) ;
#3028=CARTESIAN_POINT ( 'NONE',  ( 0.9996874511566293808, -39.97499999999999432, -9.000000000000000000 ) ) ;
#3032=VERTEX_POINT ( 'NONE', #13400 ) ;
#3041=CIRCLE ( 'NONE', #18383, 5.000000000000000888 ) ;
#3044=PRODUCT_DEFINITION_CONTEXT ( 'detailed design', #11656, 'design' ) ;
#3057=EDGE_CURVE ( 'NONE', #9040, #13819, #753, .T. ) ;
#3067=AXIS2_PLACEMENT_3D ( 'NONE', #14328, #11584, #15815 ) ;
#3068=ADVANCED_FACE ( 'NONE', ( #10831 ), #18798, .F. ) ;
#3071=EDGE_CURVE ( 'NONE', #16560, #9875, #17124, .T. ) ;
#3084=ORIENTED_EDGE ( 'NONE', *, *, #19242, .T. ) ;
#3087=VERTEX_POINT ( 'NONE', #15643 ) ;
#3094=DIRECTION ( 'NONE',  ( -0.000000000000000000, -0.000000000000000000, 1.000000000000000000 ) ) ;
#3103=STYLED_ITEM ( 'NONE', ( #6949 ), #11988 ) ;
#3106=ORIENTED_EDGE ( 'NONE', *, *, #15806, .T. ) ;
#3109=EDGE_LOOP ( 'NONE', ( #11397, #15758, #16976, #14277 ) ) ;
#3114=ORIENTED_EDGE ( 'NONE', *, *, #1758, .F. ) ;
#3115=FACE_OUTER_BOUND ( 'NONE', #4698, .T. ) ;
#3117=DIRECTION ( 'NONE',  ( 0.000000000000000000, 0.000000000000000000, 1.000000000000000000 ) ) ;
#3118=ORIENTED_EDGE ( 'NONE', *, *, #5317, .F. ) ;
#3139=CARTESIAN_POINT ( 'NONE',  ( 4.898587196589413026E-15, -40.00000000000000000, -9.000000000000000000 ) ) ;
#3143=ORIENTED_EDGE ( 'NONE', *, *, #16372, .T. ) ;
#3155=AXIS2_PLACEMENT_3D ( 'NONE', #2176, #6298, #18271 ) ;
#3179=CARTESIAN_POINT ( 'NONE',  ( 5.130877905917420101, -39.33065161639846252, 0.000000000000000000 ) ) ;
#3183=AXIS2_PLACEMENT_3D ( 'NONE', #15961, #8694, #7029 ) ;
#3189=CARTESIAN_POINT ( 'NONE',  ( -17.32050807568872841, -30.00000000000008171, -9.000000000000000000 ) ) ;
#3195=FACE_OUTER_BOUND ( 'NONE', #4798, .T. ) ;
#3218=DIRECTION ( 'NONE',  ( 0.000000000000000000, -0.000000000000000000, 1.000000000000000000 ) ) ;
#3224=AXIS2_PLACEMENT_3D ( 'NONE', #16140, #8671, #14643 ) ;
#3227=ADVANCED_FACE ( 'NONE', ( #19092 ), #5347, .T. ) ;
#3234=DIRECTION ( 'NONE',  ( 0.000000000000000000, 0.000000000000000000, 1.000000000000000000 ) ) ;
#3235=VERTEX_POINT ( 'NONE', #16137 ) ;
#3251=DIRECTION ( 'NONE',  ( -0.000000000000000000, -0.000000000000000000, -1.000000000000000000 ) ) ;
#3252=CARTESIAN_POINT ( 'NONE',  ( -18.89043790736545603, -22.09056926535314602, -9.000000000000000000 ) ) ;
#3259=CARTESIAN_POINT ( 'NONE',  ( 17.79870116617236420, -10.87825472854593301, -9.000000000000000000 ) ) ;
#3262=DIRECTION ( 'NONE',  ( -0.000000000000000000, -0.000000000000000000, 1.000000000000000000 ) ) ;
#3265=CYLINDRICAL_SURFACE ( 'NONE', #4737, 1.000000000000000000 ) ;
#3273=CYLINDRICAL_SURFACE ( 'NONE', #15867, 1.000000000000000000 ) ;
#3277=CYLINDRICAL_SURFACE ( 'NONE', #18570, 1.000000000000000888 ) ;
#3289=EDGE_CURVE ( 'NONE', #14650, #3573, #19196, .T. ) ;
#3290=ORIENTED_EDGE ( 'NONE', *, *, #9510, .F. ) ;
#3306=VECTOR ( 'NONE', #403, 1000.000000000000000 ) ;
#3310=ADVANCED_FACE ( 'NONE', ( #17904, #16624 ), #18096, .F. ) ;
#3315=DIRECTION ( 'NONE',  ( 0.000000000000000000, 0.000000000000000000, 1.000000000000000000 ) ) ;
#3320=CIRCLE ( 'NONE', #1129, 1.000000000000001110 ) ;
#3325=AXIS2_PLACEMENT_3D ( 'NONE', #14873, #8803, #1355 ) ;
#3333=AXIS2_PLACEMENT_3D ( 'NONE', #14589, #19138, #8816 ) ;
#3339=VERTEX_POINT ( 'NONE', #2903 ) ;
#3345=ORIENTED_EDGE ( 'NONE', *, *, #9091, .T. ) ;
#3361=LINE ( 'NONE', #3179, #5338 ) ;
#3362=VERTEX_POINT ( 'NONE', #10425 ) ;
#3363=AXIS2_PLACEMENT_3D ( 'NONE', #11287, #9717, #17294 ) ;
#3365=CIRCLE ( 'NONE', #1492, 20.00000000000000000 ) ;
#3378=AXIS2_PLACEMENT_3D ( 'NONE', #5893, #11859, #8924 ) ;
#3380=VECTOR ( 'NONE', #10522, 1000.000000000000000 ) ;
#3388=ORIENTED_EDGE ( 'NONE', *, *, #9768, .F. ) ;
#3395=EDGE_LOOP ( 'NONE', ( #543, #12816, #15148, #9107 ) ) ;
#3400=CARTESIAN_POINT ( 'NONE',  ( 9.037824375505689289, -37.84146099840243949, -9.000000000000000000 ) ) ;
#3404=EDGE_CURVE ( 'NONE', #19012, #11405, #2323, .T. ) ;
#3423=EDGE_CURVE ( 'NONE', #3696, #8654, #18928, .T. ) ;
#3424=CIRCLE ( 'NONE', #2180, 1.000000000000000222 ) ;
#3425=CARTESIAN_POINT ( 'NONE',  ( -19.30627432446643610, -25.22185519795866782, 0.000000000000000000 ) ) ;
#3427=CARTESIAN_POINT ( 'NONE',  ( -7.211304515372694901, -1.345319965580611843, 0.000000000000000000 ) ) ;
#3442=CIRCLE ( 'NONE', #15964, 20.00000000000000000 ) ;
#3444=ORIENTED_EDGE ( 'NONE', *, *, #9373, .F. ) ;
#3451=LINE ( 'NONE', #7942, #3901 ) ;
#3457=EDGE_CURVE ( 'NONE', #12327, #8171, #7006, .T. ) ;
#3463=CIRCLE ( 'NONE', #13479, 20.00000000000000000 ) ;
#3470=DIRECTION ( 'NONE',  ( 0.000000000000000000, 0.000000000000000000, 1.000000000000000000 ) ) ;
#3473=CARTESIAN_POINT ( 'NONE',  ( 9.037824375505316254, -2.158539001597377105, -9.000000000000000000 ) ) ;
#3478=CIRCLE ( 'NONE', #972, 1.000000000000000000 ) ;
#3481=AXIS2_PLACEMENT_3D ( 'NONE', #13077, #8268, #7092 ) ;
#3502=DIRECTION ( 'NONE',  ( -0.000000000000000000, -0.000000000000000000, 1.000000000000000000 ) ) ;
#3507=VERTEX_POINT ( 'NONE', #15228 ) ;
#3514=DIRECTION ( 'NONE',  ( -0.8090169943749487835, 0.5877852522924713607, 0.000000000000000000 ) ) ;
#3535=VERTEX_POINT ( 'NONE', #3473 ) ;
#3536=FACE_OUTER_BOUND ( 'NONE', #10820, .T. ) ;
#3538=LINE ( 'NONE', #6663, #16611 ) ;
#3545=DIRECTION ( 'NONE',  ( 0.6691306063588675634, -0.7431448254773859174, 0.000000000000000000 ) ) ;
#3552=DIRECTION ( 'NONE',  ( 0.9781476007338083534, -0.2079116908177467693, 0.000000000000000000 ) ) ;
#3553=VERTEX_POINT ( 'NONE', #2298 ) ;
#3559=CARTESIAN_POINT ( 'NONE',  ( 0.9996874511566102850, -0.02500000000000036915, -9.000000000000000000 ) ) ;
#3563=DIRECTION ( 'NONE',  ( -1.000000000000000000, 0.000000000000000000, 0.000000000000000000 ) ) ;
#3573=VERTEX_POINT ( 'NONE', #17007 ) ;
#3574=VERTEX_POINT ( 'NONE', #10803 ) ;
#3578=DIRECTION ( 'NONE',  ( 0.000000000000000000, -0.000000000000000000, 1.000000000000000000 ) ) ;
#3609=VERTEX_POINT ( 'NONE', #15517 ) ;
#3615=AXIS2_PLACEMENT_3D ( 'NONE', #2875, #11470, #2488 ) ;
#3617=ORIENTED_EDGE ( 'NONE', *, *, #5063, .F. ) ;
#3637=AXIS2_PLACEMENT_3D ( 'NONE', #5992, #7548, #17859 ) ;
#3646=ORIENTED_EDGE ( 'NONE', *, *, #19396, .F. ) ;
#3655=ORIENTED_EDGE ( 'NONE', *, *, #10145, .F. ) ;
#3668=ORIENTED_EDGE ( 'NONE', *, *, #6393, .T. ) ;
#3672=ORIENTED_EDGE ( 'NONE', *, *, #13945, .T. ) ;
#3679=EDGE_LOOP ( 'NONE', ( #13028, #5445, #10377, #12934 ) ) ;
#3680=AXIS2_PLACEMENT_3D ( 'NONE', #1496, #7469, #17980 ) ;
#3683=CIRCLE ( 'NONE', #11491, 1.000000000000000444 ) ;
#3687=VECTOR ( 'NONE', #3502, 1000.000000000000000 ) ;
#3693=ORIENTED_EDGE ( 'NONE', *, *, #9073, .F. ) ;
#3696=VERTEX_POINT ( 'NONE', #1105 ) ;
#3702=DIRECTION ( 'NONE',  ( 0.000000000000000000, -0.000000000000000000, 1.000000000000000000 ) ) ;
#3713=CIRCLE ( 'NONE', #7462, 20.00000000000000000 ) ;
#3714=AXIS2_PLACEMENT_3D ( 'NONE', #14584, #5179, #776 ) ;
#3718=ORIENTED_EDGE ( 'NONE', *, *, #17333, .F. ) ;
#3720=DIRECTION ( 'NONE',  ( 0.000000000000000000, -0.000000000000000000, 1.000000000000000000 ) ) ;
#3726=LINE ( 'NONE', #10975, #959 ) ;
#3727=VERTEX_POINT ( 'NONE', #5410 ) ;
#3728=DIRECTION ( 'NONE',  ( 0.9781476007338083534, -0.2079116908177467693, 0.000000000000000000 ) ) ;
#3732=DIRECTION ( 'NONE',  ( 0.000000000000000000, -0.000000000000000000, 1.000000000000000000 ) ) ;
#3752=VERTEX_POINT ( 'NONE', #910 ) ;
#3753=DIRECTION ( 'NONE',  ( 0.000000000000000000, 0.000000000000000000, 1.000000000000000000 ) ) ;
#3757=DIRECTION ( 'NONE',  ( 0.4999999999999974465, 0.8660254037844401509, 0.000000000000000000 ) ) ;
#3775=CARTESIAN_POINT ( 'NONE',  ( -10.93224627749297362, -36.74771600333134813, -9.000000000000000000 ) ) ;
#3784=CIRCLE ( 'NONE', #11592, 1.000000000000001110 ) ;
#3790=AXIS2_PLACEMENT_3D ( 'NONE', #11602, #3871, #14247 ) ;
#3801=ORIENTED_EDGE ( 'NONE', *, *, #6851, .F. ) ;
#3804=AXIS2_PLACEMENT_3D ( 'NONE', #16960, #2349, #858 ) ;
#3816=ADVANCED_FACE ( 'NONE', ( #17489 ), #8552, .F. ) ;
#3822=ORIENTED_EDGE ( 'NONE', *, *, #1758, .T. ) ;
#3825=( NAMED_UNIT ( * ) PLANE_ANGLE_UNIT ( ) SI_UNIT ( $, .RADIAN. ) );
#3827=LINE ( 'NONE', #13126, #2151 ) ;
#3835=FACE_OUTER_BOUND ( 'NONE', #14022, .T. ) ;
#3862=DIRECTION ( 'NONE',  ( 0.4999999999999974465, 0.8660254037844401509, 0.000000000000000000 ) ) ;
#3871=DIRECTION ( 'NONE',  ( 0.000000000000000000, 0.000000000000000000, 1.000000000000000000 ) ) ;
#3890=DIRECTION ( 'NONE',  ( 1.000000000000000000, 0.000000000000000000, 0.000000000000000000 ) ) ;
#3892=ADVANCED_FACE ( 'NONE', ( #14919 ), #19367, .F. ) ;
#3900=ORIENTED_EDGE ( 'NONE', *, *, #4144, .T. ) ;
#3901=VECTOR ( 'NONE', #7855, 1000.000000000000000 ) ;
#3902=DIRECTION ( 'NONE',  ( 1.000000000000000000, 0.000000000000000000, 0.000000000000000000 ) ) ;
#3903=EDGE_CURVE ( 'NONE', #8366, #7648, #8936, .T. ) ;
#3904=EDGE_CURVE ( 'NONE', #5077, #8618, #6388, .T. ) ;
#3905=ORIENTED_EDGE ( 'NONE', *, *, #2081, .F. ) ;
#3909=CYLINDRICAL_SURFACE ( 'NONE', #18400, 1.000000000000000888 ) ;
#3918=CARTESIAN_POINT ( 'NONE',  ( 2.449293598294706513E-15, -20.00000000000000000, -9.000000000000000000 ) ) ;
#3921=LINE ( 'NONE', #8614, #1185 ) ;
#3925=AXIS2_PLACEMENT_3D ( 'NONE', #7852, #408, #8133 ) ;
#3928=AXIS2_PLACEMENT_3D ( 'NONE', #14872, #14970, #7329 ) ;
#3941=ADVANCED_FACE ( 'NONE', ( #4444 ), #10404, .F. ) ;
#3972=ORIENTED_EDGE ( 'NONE', *, *, #12047, .F. ) ;
#3977=LINE ( 'NONE', #1331, #6648 ) ;
#3987=ORIENTED_EDGE ( 'NONE', *, *, #5991, .T. ) ;
#3992=CIRCLE ( 'NONE', #5882, 1.000000000000000666 ) ;
#3995=CARTESIAN_POINT ( 'NONE',  ( -15.51323935927264941, -32.62297130559655045, 0.000000000000000000 ) ) ;
#3997=VERTEX_POINT ( 'NONE', #121 ) ;
#3999=VERTEX_POINT ( 'NONE', #18072 ) ;
#4002=CARTESIAN_POINT ( 'NONE',  ( -9.037824375505429941, -37.84146099840256738, 0.000000000000000000 ) ) ;
#4014=DIRECTION ( 'NONE',  ( 0.000000000000000000, 0.000000000000000000, -1.000000000000000000 ) ) ;
#4020=EDGE_CURVE ( 'NONE', #18532, #4549, #3451, .T. ) ;
#4029=LINE ( 'NONE', #14207, #7447 ) ;
#4037=CIRCLE ( 'NONE', #10292, 1.000000000000000444 ) ;
#4038=VECTOR ( 'NONE', #17718, 1000.000000000000000 ) ;
#4041=FACE_BOUND ( 'NONE', #13319, .T. ) ;
#4051=AXIS2_PLACEMENT_3D ( 'NONE', #6606, #2310, #5229 ) ;
#4076=EDGE_CURVE ( 'NONE', #11041, #10947, #145, .T. ) ;
#4085=DIRECTION ( 'NONE',  ( 0.000000000000000000, 0.000000000000000000, 1.000000000000000000 ) ) ;
#4093=ORIENTED_EDGE ( 'NONE', *, *, #8697, .F. ) ;
#4094=DIRECTION ( 'NONE',  ( -0.6691306063588624564, 0.7431448254773903583, 0.000000000000000000 ) ) ;
#4096=CIRCLE ( 'NONE', #10333, 1.000000000000000000 ) ;
#4100=CARTESIAN_POINT ( 'NONE',  ( 1.000000000000000000, -14.00000000000000000, 8.999999999999998224 ) ) ;
#4105=FACE_OUTER_BOUND ( 'NONE', #8096, .T. ) ;
#4107=CARTESIAN_POINT ( 'NONE',  ( 19.30627432446651426, -25.22185519795840136, 9.000000000000000000 ) ) ;
#4120=CYLINDRICAL_SURFACE ( 'NONE', #12535, 20.00000000000000000 ) ;
#4121=CARTESIAN_POINT ( 'NONE',  ( -16.79901371501580698, -30.85325472854621864, 9.000000000000000000 ) ) ;
#4122=AXIS2_PLACEMENT_3D ( 'NONE', #7420, #3017, #1736 ) ;
#4124=CARTESIAN_POINT ( 'NONE',  ( 2.449293598294706513E-15, -20.00000000000000000, 9.000000000000000000 ) ) ;
#4126=CARTESIAN_POINT ( 'NONE',  ( -17.79870116617242459, -29.12174527145394265, 9.000000000000000000 ) ) ;
#4127=CIRCLE ( 'NONE', #15087, 1.000000000000001110 ) ;
#4135=CARTESIAN_POINT ( 'NONE',  ( -8.134732861516020819, -1.729090847147989773, -9.000000000000000000 ) ) ;
#4140=LINE ( 'NONE', #10106, #2374 ) ;
#4142=VECTOR ( 'NONE', #3218, 1000.000000000000000 ) ;
#4144=EDGE_CURVE ( 'NONE', #7961, #11553, #15209, .T. ) ;
#4148=VERTEX_POINT ( 'NONE', #3259 ) ;
#4150=CYLINDRICAL_SURFACE ( 'NONE', #3067, 1.000000000000000000 ) ;
#4153=FACE_OUTER_BOUND ( 'NONE', #6701, .T. ) ;
#4158=ORIENTED_EDGE ( 'NONE', *, *, #18214, .F. ) ;
#4159=ORIENTED_EDGE ( 'NONE', *, *, #19179, .T. ) ;
#4167=ORIENTED_EDGE ( 'NONE', *, *, #14666, .T. ) ;
#4171=ADVANCED_FACE ( 'NONE', ( #3835 ), #11163, .F. ) ;
#4176=CARTESIAN_POINT ( 'NONE',  ( 1.000000000000000444, -15.10102051443364246, 9.000000000000000000 ) ) ;
#4192=VERTEX_POINT ( 'NONE', #5393 ) ;
#4197=CARTESIAN_POINT ( 'NONE',  ( -11.75570504584948139, -3.819660112501066518, -9.000000000000000000 ) ) ;
#4198=LINE ( 'NONE', #11731, #5821 ) ;
#4199=CARTESIAN_POINT ( 'NONE',  ( 2.449293598294706513E-15, -20.00000000000000000, -9.000000000000000000 ) ) ;
#4202=VERTEX_POINT ( 'NONE', #17276 ) ;
#4210=ORIENTED_EDGE ( 'NONE', *, *, #6749, .F. ) ;
#4218=CARTESIAN_POINT ( 'NONE',  ( 4.898587196589413026E-15, -40.00000000000000000, -9.000000000000000000 ) ) ;
#4227=EDGE_LOOP ( 'NONE', ( #7212, #14533, #8791, #5951 ) ) ;
#4231=DIRECTION ( 'NONE',  ( 1.000000000000000000, 0.000000000000000000, 0.000000000000000000 ) ) ;
#4234=CARTESIAN_POINT ( 'NONE',  ( -16.79901371501587803, -9.146745271453902149, 9.000000000000000000 ) ) ;
#4256=EDGE_CURVE ( 'NONE', #4327, #16340, #16088, .T. ) ;
#4270=CIRCLE ( 'NONE', #18683, 5.000000000000000888 ) ;
#4274=ORIENTED_EDGE ( 'NONE', *, *, #6301, .T. ) ;
#4287=CARTESIAN_POINT ( 'NONE',  ( 3.175194142252359963, -39.74634503291702003, 9.000000000000000000 ) ) ;
#4290=VECTOR ( 'NONE', #11440, 1000.000000000000000 ) ;
#4292=FACE_OUTER_BOUND ( 'NONE', #9984, .T. ) ;
#4293=ADVANCED_FACE ( 'NONE', ( #5588 ), #17570, .T. ) ;
#4294=LINE ( 'NONE', #4396, #18550 ) ;
#4302=CIRCLE ( 'NONE', #7743, 20.00000000000000000 ) ;
#4310=CARTESIAN_POINT ( 'NONE',  ( 0.000000000000000000, 0.000000000000000000, 9.000000000000000000 ) ) ;
#4314=DIRECTION ( 'NONE',  ( -0.1045284632676425907, -0.9945218953682745111, 0.000000000000000000 ) ) ;
#4315=VECTOR ( 'NONE', #11465, 1000.000000000000000 ) ;
#4319=AXIS2_PLACEMENT_3D ( 'NONE', #10138, #9942, #8674 ) ;
#4327=VERTEX_POINT ( 'NONE', #7638 ) ;
#4332=CARTESIAN_POINT ( 'NONE',  ( 2.449293598294706513E-15, -20.00000000000000000, 15.00000000000000355 ) ) ;
#4342=AXIS2_PLACEMENT_3D ( 'NONE', #6725, #5158, #8201 ) ;
#4343=CARTESIAN_POINT ( 'NONE',  ( -16.32050807568879236, -10.00000000000004263, 9.000000000000000000 ) ) ;
#4346=ORIENTED_EDGE ( 'NONE', *, *, #16482, .T. ) ;
#4350=EDGE_CURVE ( 'NONE', #7750, #15438, #8291, .T. ) ;
#4352=CARTESIAN_POINT ( 'NONE',  ( 14.86289650954772590, -6.617387872822656725, -9.000000000000000000 ) ) ;
#4353=AXIS2_PLACEMENT_3D ( 'NONE', #7604, #17635, #7218 ) ;
#4354=VECTOR ( 'NONE', #17310, 1000.000000000000000 ) ;
#4359=CARTESIAN_POINT ( 'NONE',  ( 2.449293598294706513E-15, -20.00000000000000000, -9.000000000000000000 ) ) ;
#4370=CYLINDRICAL_SURFACE ( 'NONE', #16297, 1.000000000000000000 ) ;
#4375=ADVANCED_FACE ( 'NONE', ( #10572 ), #2860, .T. ) ;
#4378=ORIENTED_EDGE ( 'NONE', *, *, #9501, .F. ) ;
#4381=CIRCLE ( 'NONE', #15970, 0.9999999999999980016 ) ;
#4383=CARTESIAN_POINT ( 'NONE',  ( -17.32050807568872841, -30.00000000000008171, -9.000000000000000000 ) ) ;
#4386=CYLINDRICAL_SURFACE ( 'NONE', #6009, 1.000000000000000888 ) ;
#4396=CARTESIAN_POINT ( 'NONE',  ( 15.51323935927282704, -32.62297130559633729, 0.000000000000000000 ) ) ;
#4397=AXIS2_PLACEMENT_3D ( 'NONE', #18806, #4085, #5643 ) ;
#4400=ORIENTED_EDGE ( 'NONE', *, *, #8738, .F. ) ;
#4406=CIRCLE ( 'NONE', #1275, 1.000000000000000222 ) ;
#4408=CARTESIAN_POINT ( 'NONE',  ( -16.32050807568872841, -30.00000000000008171, 9.000000000000000000 ) ) ;
#4413=EDGE_CURVE ( 'NONE', #4549, #17921, #16444, .T. ) ;
#4424=AXIS2_PLACEMENT_3D ( 'NONE', #17611, #18791, #11209 ) ;
#4426=AXIS2_PLACEMENT_3D ( 'NONE', #17204, #1023, #9728 ) ;
#4431=DIRECTION ( 'NONE',  ( -0.000000000000000000, -0.000000000000000000, -1.000000000000000000 ) ) ;
#4434=ORIENTED_EDGE ( 'NONE', *, *, #575, .F. ) ;
#4441=CARTESIAN_POINT ( 'NONE',  ( 16.79901371501572882, -9.146745271453649906, -9.000000000000000000 ) ) ;
#4444=FACE_OUTER_BOUND ( 'NONE', #4704, .T. ) ;
#4458=ORIENTED_EDGE ( 'NONE', *, *, #9368, .T. ) ;
#4481=ORIENTED_EDGE ( 'NONE', *, *, #14777, .F. ) ;
#4488=ORIENTED_EDGE ( 'NONE', *, *, #6281, .F. ) ;
#4500=CARTESIAN_POINT ( 'NONE',  ( 11.75570504584926468, -3.819660112500910198, -9.000000000000000000 ) ) ;
#4515=DIRECTION ( 'NONE',  ( -0.000000000000000000, 0.000000000000000000, 1.000000000000000000 ) ) ;
#4528=DIRECTION ( 'NONE',  ( -1.000000000000000000, 0.000000000000000000, 0.000000000000000000 ) ) ;
#4542=CARTESIAN_POINT ( 'NONE',  ( -10.93224627749309796, -3.252283996668732691, -9.000000000000000000 ) ) ;
#4544=EDGE_CURVE ( 'NONE', #4327, #12719, #5797, .T. ) ;
#4548=EDGE_CURVE ( 'NONE', #1857, #19012, #16768, .T. ) ;
#4549=VERTEX_POINT ( 'NONE', #9201 ) ;
#4565=AXIS2_PLACEMENT_3D ( 'NONE', #2367, #5098, #9690 ) ;
#4580=ORIENTED_EDGE ( 'NONE', *, *, #5083, .T. ) ;
#4586=CARTESIAN_POINT ( 'NONE',  ( -5.130877905917297532, -0.6693483836015048372, -9.000000000000000000 ) ) ;
#4593=ORIENTED_EDGE ( 'NONE', *, *, #4350, .F. ) ;
#4602=ORIENTED_EDGE ( 'NONE', *, *, #17189, .T. ) ;
#4639=DIRECTION ( 'NONE',  ( -0.000000000000000000, 0.000000000000000000, -1.000000000000000000 ) ) ;
#4646=AXIS2_PLACEMENT_3D ( 'NONE', #13540, #4431, #4528 ) ;
#4655=DIRECTION ( 'NONE',  ( 0.000000000000000000, 0.000000000000000000, 1.000000000000000000 ) ) ;
#4661=DIRECTION ( 'NONE',  ( 0.000000000000000000, 0.000000000000000000, 1.000000000000000000 ) ) ;
#4670=CYLINDRICAL_SURFACE ( 'NONE', #8743, 1.000000000000000888 ) ;
#4678=CYLINDRICAL_SURFACE ( 'NONE', #12220, 1.000000000000000888 ) ;
#4683=DIRECTION ( 'NONE',  ( 1.000000000000000000, 0.000000000000000000, 0.000000000000000000 ) ) ;
#4698=EDGE_LOOP ( 'NONE', ( #11796, #16545, #10726, #5768 ) ) ;
#4699=DIRECTION ( 'NONE',  ( -0.9135454576426043083, 0.4067366430757925477, 0.000000000000000000 ) ) ;
#4704=EDGE_LOOP ( 'NONE', ( #4813, #15884, #2162, #16622 ) ) ;
#4709=AXIS2_PLACEMENT_3D ( 'NONE', #12386, #437, #6406 ) ;
#4723=DIRECTION ( 'NONE',  ( 0.000000000000000000, 0.000000000000000000, 1.000000000000000000 ) ) ;
#4724=ADVANCED_FACE ( 'NONE', ( #4105 ), #864, .T. ) ;
#4731=CIRCLE ( 'NONE', #6913, 20.00000000000000000 ) ;
#4733=EDGE_CURVE ( 'NONE', #7722, #4891, #18958, .T. ) ;
#4737=AXIS2_PLACEMENT_3D ( 'NONE', #327, #16997, #10889 ) ;
#4744=VECTOR ( 'NONE', #9385, 1000.000000000000000 ) ;
#4767=VERTEX_POINT ( 'NONE', #6650 ) ;
#4771=ORIENTED_EDGE ( 'NONE', *, *, #12858, .F. ) ;
#4778=CYLINDRICAL_SURFACE ( 'NONE', #12324, 1.000000000000000000 ) ;
#4788=EDGE_CURVE ( 'NONE', #15338, #5469, #7034, .T. ) ;
#4795=FACE_OUTER_BOUND ( 'NONE', #17846, .T. ) ;
#4797=DIRECTION ( 'NONE',  ( 0.000000000000000000, 0.000000000000000000, 1.000000000000000000 ) ) ;
#4798=EDGE_LOOP ( 'NONE', ( #13012, #17902, #9560, #10457 ) ) ;
#4800=VERTEX_POINT ( 'NONE', #8217 ) ;
#4812=FACE_OUTER_BOUND ( 'NONE', #6564, .T. ) ;
#4813=ORIENTED_EDGE ( 'NONE', *, *, #15484, .F. ) ;
#4821=VECTOR ( 'NONE', #4639, 1000.000000000000000 ) ;
#4823=CARTESIAN_POINT ( 'NONE',  ( -17.79870116617242459, -29.12174527145394265, -9.000000000000000000 ) ) ;
#4837=CARTESIAN_POINT ( 'NONE',  ( 10.93224627749321876, -36.74771600333119181, -9.000000000000000000 ) ) ;
#4845=DIRECTION ( 'NONE',  ( -0.000000000000000000, 0.000000000000000000, -1.000000000000000000 ) ) ;
#4860=ADVANCED_FACE ( 'NONE', ( #4292 ), #16363, .F. ) ;
#4861=ORIENTED_EDGE ( 'NONE', *, *, #16482, .F. ) ;
#4862=CIRCLE ( 'NONE', #3928, 0.9999999999999995559 ) ;
#4867=DIRECTION ( 'NONE',  ( 0.000000000000000000, 0.000000000000000000, 1.000000000000000000 ) ) ;
#4889=ORIENTED_EDGE ( 'NONE', *, *, #13719, .T. ) ;
#4891=VERTEX_POINT ( 'NONE', #13115 ) ;
#4945=ORIENTED_EDGE ( 'NONE', *, *, #4350, .T. ) ;
#4947=EDGE_CURVE ( 'NONE', #14568, #2854, #4862, .T. ) ;
#4949=VECTOR ( 'NONE', #8120, 1000.000000000000000 ) ;
#4959=EDGE_CURVE ( 'NONE', #5570, #13074, #17398, .T. ) ;
#4963=CARTESIAN_POINT ( 'NONE',  ( 19.30627432446651426, -25.22185519795840136, 0.000000000000000000 ) ) ;
#4965=ORIENTED_EDGE ( 'NONE', *, *, #16830, .F. ) ;
#4972=ORIENTED_EDGE ( 'NONE', *, *, #1133, .T. ) ;
#4979=CIRCLE ( 'NONE', #18465, 1.000000000000000222 ) ;
#4981=CARTESIAN_POINT ( 'NONE',  ( -18.02113032590308705, -13.81966011250110249, 9.000000000000000000 ) ) ;
#4995=ORIENTED_EDGE ( 'NONE', *, *, #11347, .T. ) ;
#5014=DIRECTION ( 'NONE',  ( 0.000000000000000000, 0.000000000000000000, 1.000000000000000000 ) ) ;
#5022=CIRCLE ( 'NONE', #6584, 0.9999999999999995559 ) ;
#5027=CARTESIAN_POINT ( 'NONE',  ( 8.134732861515777458, -1.729090847147875198, -9.000000000000000000 ) ) ;
#5033=DIRECTION ( 'NONE',  ( -0.000000000000000000, -0.000000000000000000, -1.000000000000000000 ) ) ;
#5036=AXIS2_PLACEMENT_3D ( 'NONE', #9411, #12839, #3728 ) ;
#5046=CARTESIAN_POINT ( 'NONE',  ( -12.54977455159113653, -35.57251292194792569, 0.000000000000000000 ) ) ;
#5048=DIRECTION ( 'NONE',  ( 0.000000000000000000, 0.000000000000000000, 1.000000000000000000 ) ) ;
#5063=EDGE_CURVE ( 'NONE', #9040, #4202, #438, .T. ) ;
#5070=AXIS2_PLACEMENT_3D ( 'NONE', #7133, #12648, #16161 ) ;
#5071=DIRECTION ( 'NONE',  ( -0.000000000000000000, 0.000000000000000000, 1.000000000000000000 ) ) ;
#5077=VERTEX_POINT ( 'NONE', #520 ) ;
#5082=CARTESIAN_POINT ( 'NONE',  ( 12.54977455159103705, -4.427487078051979275, 0.000000000000000000 ) ) ;
#5083=EDGE_CURVE ( 'NONE', #18931, #12414, #7324, .T. ) ;
#5092=ORIENTED_EDGE ( 'NONE', *, *, #2928, .F. ) ;
#5095=DIRECTION ( 'NONE',  ( 0.000000000000000000, 0.000000000000000000, 1.000000000000000000 ) ) ;
#5098=DIRECTION ( 'NONE',  ( 0.000000000000000000, 0.000000000000000000, 1.000000000000000000 ) ) ;
#5105=CARTESIAN_POINT ( 'NONE',  ( -0.9996874511566050669, -39.97499999999999432, 0.000000000000000000 ) ) ;
#5111=CARTESIAN_POINT ( 'NONE',  ( 5.130877905917027526, -0.6693483836014323396, -9.000000000000000000 ) ) ;
#5113=ORIENTED_EDGE ( 'NONE', *, *, #9863, .T. ) ;
#5158=DIRECTION ( 'NONE',  ( 0.000000000000000000, 0.000000000000000000, 1.000000000000000000 ) ) ;
#5161=CARTESIAN_POINT ( 'NONE',  ( -18.89043790736547379, -17.90943073464699609, -9.000000000000000000 ) ) ;
#5165=ORIENTED_EDGE ( 'NONE', *, *, #4413, .F. ) ;
#5167=ORIENTED_EDGE ( 'NONE', *, *, #15756, .F. ) ;
#5168=EDGE_CURVE ( 'NONE', #4549, #9525, #14205, .T. ) ;
#5174=CARTESIAN_POINT ( 'NONE',  ( -11.75570504584948139, -3.819660112501066518, 9.000000000000000000 ) ) ;
#5179=DIRECTION ( 'NONE',  ( -0.000000000000000000, -0.000000000000000000, -1.000000000000000000 ) ) ;
#5180=AXIS2_PLACEMENT_3D ( 'NONE', #12629, #17546, #18925 ) ;
#5182=ADVANCED_FACE ( 'NONE', ( #8058 ), #14231, .F. ) ;
#5184=DIRECTION ( 'NONE',  ( -0.000000000000000000, -0.000000000000000000, -1.000000000000000000 ) ) ;
#5186=ORIENTED_EDGE ( 'NONE', *, *, #19179, .F. ) ;
#5192=ADVANCED_FACE ( 'NONE', ( #4153 ), #10117, .F. ) ;
#5204=AXIS2_PLACEMENT_3D ( 'NONE', #13538, #12059, #15001 ) ;
#5207=CYLINDRICAL_SURFACE ( 'NONE', #7191, 20.00000000000000000 ) ;
#5229=DIRECTION ( 'NONE',  ( 1.000000000000000000, 0.000000000000000000, 0.000000000000000000 ) ) ;
#5247=CARTESIAN_POINT ( 'NONE',  ( 0.9996874511566102850, -0.02500000000000036915, 0.000000000000000000 ) ) ;
#5253=DIRECTION ( 'NONE',  ( 1.000000000000000000, 0.000000000000000000, 0.000000000000000000 ) ) ;
#5260=AXIS2_PLACEMENT_3D ( 'NONE', #4135, #8633, #2679 ) ;
#5267=EDGE_LOOP ( 'NONE', ( #14667, #16805, #5651, #17818 ) ) ;
#5280=ORIENTED_EDGE ( 'NONE', *, *, #11285, .T. ) ;
#5282=( LENGTH_UNIT ( ) NAMED_UNIT ( * ) SI_UNIT ( .MILLI., .METRE. ) );
#5286=DIRECTION ( 'NONE',  ( -0.000000000000000000, -0.000000000000000000, 1.000000000000000000 ) ) ;
#5294=DIRECTION ( 'NONE',  ( -0.000000000000000000, 0.000000000000000000, 1.000000000000000000 ) ) ;
#5304=PRODUCT_DEFINITION ( 'UNKNOWN', '', #11035, #3044 ) ;
#5317=EDGE_CURVE ( 'NONE', #1251, #6799, #2660, .T. ) ;
#5319=AXIS2_PLACEMENT_3D ( 'NONE', #747, #5444, #5253 ) ;
#5327=EDGE_CURVE ( 'NONE', #16340, #5943, #7644, .T. ) ;
#5331=CIRCLE ( 'NONE', #5657, 0.9999999999999993339 ) ;
#5333=EDGE_LOOP ( 'NONE', ( #6052, #11619, #8224, #15688 ) ) ;
#5338=VECTOR ( 'NONE', #18186, 1000.000000000000000 ) ;
#5340=LINE ( 'NONE', #2517, #6293 ) ;
#5347=CYLINDRICAL_SURFACE ( 'NONE', #5755, 20.00000000000000000 ) ;
#5350=DIRECTION ( 'NONE',  ( 1.000000000000000000, 0.000000000000000000, 0.000000000000000000 ) ) ;
#5356=DIRECTION ( 'NONE',  ( 1.000000000000000000, 0.000000000000000000, 0.000000000000000000 ) ) ;
#5364=ORIENTED_EDGE ( 'NONE', *, *, #2247, .F. ) ;
#5365=AXIS2_PLACEMENT_3D ( 'NONE', #8165, #6792, #3862 ) ;
#5367=DIRECTION ( 'NONE',  ( 1.000000000000000000, 0.000000000000000000, 0.000000000000000000 ) ) ;
#5380=CIRCLE ( 'NONE', #18853, 20.00000000000000000 ) ;
#5382=ORIENTED_EDGE ( 'NONE', *, *, #14903, .F. ) ;
#5387=ORIENTED_EDGE ( 'NONE', *, *, #17679, .F. ) ;
#5393=CARTESIAN_POINT ( 'NONE',  ( -17.79870116617249209, -10.87825472854619413, -9.000000000000000000 ) ) ;
#5410=CARTESIAN_POINT ( 'NONE',  ( -19.76107906696391225, -16.91783288752853665, 9.000000000000000000 ) ) ;
#5411=EDGE_CURVE ( 'NONE', #13074, #3032, #8939, .T. ) ;
#5427=DIRECTION ( 'NONE',  ( 1.000000000000000000, 0.000000000000000000, 0.000000000000000000 ) ) ;
#5434=EDGE_CURVE ( 'NONE', #337, #11695, #14922, .T. ) ;
#5439=LINE ( 'NONE', #14644, #18733 ) ;
#5444=DIRECTION ( 'NONE',  ( 0.000000000000000000, 0.000000000000000000, 1.000000000000000000 ) ) ;
#5445=ORIENTED_EDGE ( 'NONE', *, *, #6064, .T. ) ;
#5458=DIRECTION ( 'NONE',  ( -0.000000000000000000, 0.000000000000000000, 1.000000000000000000 ) ) ;
#5460=LINE ( 'NONE', #8598, #12249 ) ;
#5465=DIRECTION ( 'NONE',  ( -0.000000000000000000, -0.000000000000000000, -1.000000000000000000 ) ) ;
#5467=CARTESIAN_POINT ( 'NONE',  ( -4.158233816355195955, -0.4370479853238878887, 9.000000000000000000 ) ) ;
#5469=VERTEX_POINT ( 'NONE', #1600 ) ;
#5470=ORIENTED_EDGE ( 'NONE', *, *, #18391, .T. ) ;
#5473=DIRECTION ( 'NONE',  ( 0.1045284632676494602, 0.9945218953682738450, 0.000000000000000000 ) ) ;
#5474=DIRECTION ( 'NONE',  ( 1.000000000000000000, 0.000000000000000000, 0.000000000000000000 ) ) ;
#5500=AXIS2_PLACEMENT_3D ( 'NONE', #16670, #13317, #95 ) ;
#5505=FACE_OUTER_BOUND ( 'NONE', #17220, .T. ) ;
#5514=FACE_OUTER_BOUND ( 'NONE', #3395, .T. ) ;
#5517=ORIENTED_EDGE ( 'NONE', *, *, #14535, .F. ) ;
#5549=ORIENTED_EDGE ( 'NONE', *, *, #6162, .T. ) ;
#5551=LINE ( 'NONE', #958, #18374 ) ;
#5552=ADVANCED_FACE ( 'NONE', ( #2886 ), #14822, .F. ) ;
#5553=AXIS2_PLACEMENT_3D ( 'NONE', #12657, #12456, #8041 ) ;
#5556=ORIENTED_EDGE ( 'NONE', *, *, #6027, .F. ) ;
#5570=VERTEX_POINT ( 'NONE', #17083 ) ;
#5580=CARTESIAN_POINT ( 'NONE',  ( -8.134732861515892921, -38.27090915285207018, 9.000000000000000000 ) ) ;
#5581=ORIENTED_EDGE ( 'NONE', *, *, #13341, .F. ) ;
#5584=VECTOR ( 'NONE', #15364, 1000.000000000000000 ) ;
#5585=CARTESIAN_POINT ( 'NONE',  ( -14.86289650954781649, -33.38261212717723936, -9.000000000000000000 ) ) ;
#5588=FACE_OUTER_BOUND ( 'NONE', #4227, .T. ) ;
#5596=FACE_OUTER_BOUND ( 'NONE', #12693, .T. ) ;
#5600=VERTEX_POINT ( 'NONE', #9507 ) ;
#5603=CARTESIAN_POINT ( 'NONE',  ( 19.76107906696393357, -23.08216711247132835, 9.000000000000000000 ) ) ;
#5607=DIRECTION ( 'NONE',  ( 0.000000000000000000, 0.000000000000000000, 1.000000000000000000 ) ) ;
#5620=ADVANCED_FACE ( 'NONE', ( #15406 ), #8036, .T. ) ;
#5623=ORIENTED_EDGE ( 'NONE', *, *, #16859, .F. ) ;
#5630=DIRECTION ( 'NONE',  ( -0.1045284632676563297, 0.9945218953682731788, 0.000000000000000000 ) ) ;
#5631=ORIENTED_EDGE ( 'NONE', *, *, #12974, .F. ) ;
#5636=DIRECTION ( 'NONE',  ( 0.000000000000000000, -0.000000000000000000, 1.000000000000000000 ) ) ;
#5640=CARTESIAN_POINT ( 'NONE',  ( -18.02113032590304442, -26.18033988749903074, 9.000000000000000000 ) ) ;
#5643=DIRECTION ( 'NONE',  ( 0.3090169943749456194, 0.9510565162951541973, 0.000000000000000000 ) ) ;
#5645=AXIS2_PLACEMENT_3D ( 'NONE', #11200, #9730, #9823 ) ;
#5646=ORIENTED_EDGE ( 'NONE', *, *, #13098, .T. ) ;
#5651=ORIENTED_EDGE ( 'NONE', *, *, #14442, .T. ) ;
#5652=VERTEX_POINT ( 'NONE', #8235 ) ;
#5657=AXIS2_PLACEMENT_3D ( 'NONE', #9679, #17548, #10074 ) ;
#5669=EDGE_CURVE ( 'NONE', #2657, #3339, #8139, .T. ) ;
#5671=CIRCLE ( 'NONE', #3804, 1.000000000000000666 ) ;
#5686=DIRECTION ( 'NONE',  ( 1.000000000000000000, 0.000000000000000000, 0.000000000000000000 ) ) ;
#5687=CIRCLE ( 'NONE', #19181, 1.000000000000001110 ) ;
#5688=AXIS2_PLACEMENT_3D ( 'NONE', #5905, #11874, #17883 ) ;
#5700=VERTEX_POINT ( 'NONE', #2479 ) ;
#5702=ADVANCED_FACE ( 'NONE', ( #11662 ), #2766, .F. ) ;
#5709=AXIS2_PLACEMENT_3D ( 'NONE', #16357, #16741, #10541 ) ;
#5717=CIRCLE ( 'NONE', #16051, 1.000000000000000000 ) ;
#5718=DIRECTION ( 'NONE',  ( 1.000000000000000000, 0.000000000000000000, 0.000000000000000000 ) ) ;
#5720=DIRECTION ( 'NONE',  ( 1.000000000000000000, 0.000000000000000000, 0.000000000000000000 ) ) ;
#5726=ORIENTED_EDGE ( 'NONE', *, *, #3071, .F. ) ;
#5729=CARTESIAN_POINT ( 'NONE',  ( 2.449293598294706513E-15, -20.00000000000000000, 9.000000000000000000 ) ) ;
#5731=EDGE_LOOP ( 'NONE', ( #9192, #310, #9849, #3672 ) ) ;
#5743=DIRECTION ( 'NONE',  ( 0.000000000000000000, 0.000000000000000000, 1.000000000000000000 ) ) ;
#5753=FACE_OUTER_BOUND ( 'NONE', #13702, .T. ) ;
#5755=AXIS2_PLACEMENT_3D ( 'NONE', #17515, #17707, #9938 ) ;
#5766=DIRECTION ( 'NONE',  ( 0.8090169943749546677, -0.5877852522924632561, 0.000000000000000000 ) ) ;
#5768=ORIENTED_EDGE ( 'NONE', *, *, #8194, .T. ) ;
#5779=ORIENTED_EDGE ( 'NONE', *, *, #4959, .F. ) ;
#5788=LINE ( 'NONE', #1578, #19135 ) ;
#5796=ORIENTED_EDGE ( 'NONE', *, *, #12047, .T. ) ;
#5797=CIRCLE ( 'NONE', #7347, 1.000000000000001110 ) ;
#5806=DIRECTION ( 'NONE',  ( 1.000000000000000000, 0.000000000000000000, 0.000000000000000000 ) ) ;
#5807=EDGE_CURVE ( 'NONE', #17921, #16520, #14505, .T. ) ;
#5815=CIRCLE ( 'NONE', #10194, 0.9999999999999982236 ) ;
#5818=FACE_OUTER_BOUND ( 'NONE', #5267, .T. ) ;
#5821=VECTOR ( 'NONE', #6063, 1000.000000000000000 ) ;
#5822=EDGE_CURVE ( 'NONE', #439, #8857, #18238, .T. ) ;
#5831=AXIS2_PLACEMENT_3D ( 'NONE', #11432, #11338, #4094 ) ;
#5842=CARTESIAN_POINT ( 'NONE',  ( 18.68843350152485527, -12.87662627267923909, 0.000000000000000000 ) ) ;
#5843=VECTOR ( 'NONE', #18673, 1000.000000000000000 ) ;
#5852=EDGE_CURVE ( 'NONE', #3997, #6513, #5788, .T. ) ;
#5853=ORIENTED_EDGE ( 'NONE', *, *, #2466, .F. ) ;
#5859=CARTESIAN_POINT ( 'NONE',  ( -14.17539641854921229, -5.891203581560112923, -9.000000000000000000 ) ) ;
#5870=DIRECTION ( 'NONE',  ( 1.000000000000000000, 0.000000000000000000, 0.000000000000000000 ) ) ;
#5875=EDGE_LOOP ( 'NONE', ( #114, #3822, #11936, #6807 ) ) ;
#5882=AXIS2_PLACEMENT_3D ( 'NONE', #13913, #9317, #3545 ) ;
#5891=LINE ( 'NONE', #2585, #16912 ) ;
#5893=CARTESIAN_POINT ( 'NONE',  ( 2.449293598294706513E-15, -20.00000000000000000, 9.000000000000000000 ) ) ;
#5898=CARTESIAN_POINT ( 'NONE',  ( 2.449293598294706513E-15, -20.00000000000000000, 9.000000000000000000 ) ) ;
#5902=DIRECTION ( 'NONE',  ( 0.000000000000000000, 0.000000000000000000, 1.000000000000000000 ) ) ;
#5905=CARTESIAN_POINT ( 'NONE',  ( 2.449293598294706513E-15, -20.00000000000000000, 15.00000000000000355 ) ) ;
#5926=CIRCLE ( 'NONE', #4051, 20.00000000000000000 ) ;
#5928=ORIENTED_EDGE ( 'NONE', *, *, #4733, .F. ) ;
#5941=CARTESIAN_POINT ( 'NONE',  ( 4.158233816355333623, -39.56295201467608535, -9.000000000000000000 ) ) ;
#5943=VERTEX_POINT ( 'NONE', #10676 ) ;
#5944=VECTOR ( 'NONE', #309, 1000.000000000000000 ) ;
#5946=LINE ( 'NONE', #7117, #4038 ) ;
#5947=ORIENTED_EDGE ( 'NONE', *, *, #7232, .T. ) ;
#5951=ORIENTED_EDGE ( 'NONE', *, *, #18214, .T. ) ;
#5955=DIRECTION ( 'NONE',  ( -0.000000000000000000, -0.000000000000000000, 1.000000000000000000 ) ) ;
#5958=VECTOR ( 'NONE', #16196, 1000.000000000000000 ) ;
#5961=CARTESIAN_POINT ( 'NONE',  ( -4.158233816355060064, -39.56295201467614220, -9.000000000000000000 ) ) ;
#5966=AXIS2_PLACEMENT_3D ( 'NONE', #11810, #1635, #17814 ) ;
#5972=LINE ( 'NONE', #7145, #16867 ) ;
#5986=UNCERTAINTY_MEASURE_WITH_UNIT (LENGTH_MEASURE( 1.000000000000000082E-05 ), #5282, 'distance_accuracy_value', 'NONE');
#5989=AXIS2_PLACEMENT_3D ( 'NONE', #19040, #19143, #5686 ) ;
#5991=EDGE_CURVE ( 'NONE', #585, #6953, #13484, .T. ) ;
#5992=CARTESIAN_POINT ( 'NONE',  ( -19.89043790736545603, -22.09056926535314602, -9.000000000000000000 ) ) ;
#6003=CARTESIAN_POINT ( 'NONE',  ( 7.211304515372431112, -1.345319965580505484, -9.000000000000000000 ) ) ;
#6009=AXIS2_PLACEMENT_3D ( 'NONE', #19226, #5955, #13957 ) ;
#6021=ORIENTED_EDGE ( 'NONE', *, *, #6410, .T. ) ;
#6024=DIRECTION ( 'NONE',  ( 0.000000000000000000, 0.000000000000000000, 1.000000000000000000 ) ) ;
#6026=CARTESIAN_POINT ( 'NONE',  ( 2.449293598294706513E-15, -20.00000000000000000, 15.00000000000000355 ) ) ;
#6027=EDGE_CURVE ( 'NONE', #3032, #3339, #5022, .T. ) ;
#6028=ORIENTED_EDGE ( 'NONE', *, *, #12926, .F. ) ;
#6030=ORIENTED_EDGE ( 'NONE', *, *, #7489, .F. ) ;
#6052=ORIENTED_EDGE ( 'NONE', *, *, #2938, .F. ) ;
#6063=DIRECTION ( 'NONE',  ( -0.000000000000000000, -0.000000000000000000, 1.000000000000000000 ) ) ;
#6064=EDGE_CURVE ( 'NONE', #14568, #11186, #10962, .T. ) ;
#6065=DIRECTION ( 'NONE',  ( 1.000000000000000000, 0.000000000000000000, 0.000000000000000000 ) ) ;
#6076=ORIENTED_EDGE ( 'NONE', *, *, #116, .F. ) ;
#6092=EDGE_CURVE ( 'NONE', #3574, #11553, #2848, .T. ) ;
#6094=EDGE_LOOP ( 'NONE', ( #2266, #6456, #1154, #1279 ) ) ;
#6101=DIRECTION ( 'NONE',  ( 0.000000000000000000, -0.000000000000000000, 1.000000000000000000 ) ) ;
#6104=CARTESIAN_POINT ( 'NONE',  ( -10.75570504584948139, -3.819660112501066518, -9.000000000000000000 ) ) ;
#6115=ORIENTED_EDGE ( 'NONE', *, *, #5327, .T. ) ;
#6119=ORIENTED_EDGE ( 'NONE', *, *, #14107, .T. ) ;
#6124=LINE ( 'NONE', #14943, #3380 ) ;
#6129=CARTESIAN_POINT ( 'NONE',  ( 19.97007065299863271, -21.09374499507102740, 9.000000000000000000 ) ) ;
#6138=CARTESIAN_POINT ( 'NONE',  ( 2.449293598294706513E-15, -20.00000000000000000, 9.000000000000000000 ) ) ;
#6139=ORIENTED_EDGE ( 'NONE', *, *, #3057, .T. ) ;
#6146=AXIS2_PLACEMENT_3D ( 'NONE', #8429, #14503, #1087 ) ;
#6162=EDGE_CURVE ( 'NONE', #3362, #9866, #6363, .T. ) ;
#6168=CIRCLE ( 'NONE', #13047, 0.9999999999999993339 ) ;
#6172=DIRECTION ( 'NONE',  ( -0.000000000000000000, -0.000000000000000000, 1.000000000000000000 ) ) ;
#6183=CYLINDRICAL_SURFACE ( 'NONE', #5204, 20.00000000000000000 ) ;
#6195=CARTESIAN_POINT ( 'NONE',  ( -19.02113032590304442, -26.18033988749903074, -9.000000000000000000 ) ) ;
#6196=DIRECTION ( 'NONE',  ( 1.000000000000000000, 0.000000000000000000, 0.000000000000000000 ) ) ;
#6200=CARTESIAN_POINT ( 'NONE',  ( -19.97007065299861850, -18.90625500492883759, 9.000000000000000000 ) ) ;
#6206=ORIENTED_EDGE ( 'NONE', *, *, #1633, .T. ) ;
#6214=DIRECTION ( 'NONE',  ( 1.000000000000000000, 0.000000000000000000, 0.000000000000000000 ) ) ;
#6215=EDGE_CURVE ( 'NONE', #7491, #10940, #11594, .T. ) ;
#6216=AXIS2_PLACEMENT_3D ( 'NONE', #15292, #1873, #15196 ) ;
#6221=EDGE_CURVE ( 'NONE', #6930, #508, #5331, .T. ) ;
#6227=CARTESIAN_POINT ( 'NONE',  ( -19.02113032590308705, -13.81966011250110249, -9.000000000000000000 ) ) ;
#6232=ORIENTED_EDGE ( 'NONE', *, *, #11953, .T. ) ;
#6240=CARTESIAN_POINT ( 'NONE',  ( -10.75570504584937304, -36.18033988749900942, -9.000000000000000000 ) ) ;
#6242=CARTESIAN_POINT ( 'NONE',  ( -19.30627432446643610, -25.22185519795866782, 9.000000000000000000 ) ) ;
#6246=LINE ( 'NONE', #6342, #13203 ) ;
#6248=ORIENTED_EDGE ( 'NONE', *, *, #17454, .T. ) ;
#6258=ORIENTED_EDGE ( 'NONE', *, *, #10215, .F. ) ;
#6266=DIRECTION ( 'NONE',  ( 0.000000000000000000, 0.000000000000000000, 1.000000000000000000 ) ) ;
#6272=DIRECTION ( 'NONE',  ( -1.000000000000000000, -4.082155997157843695E-16, 0.000000000000000000 ) ) ;
#6273=CIRCLE ( 'NONE', #14408, 20.00000000000000000 ) ;
#6281=EDGE_CURVE ( 'NONE', #17942, #15146, #8465, .T. ) ;
#6285=DIRECTION ( 'NONE',  ( 0.000000000000000000, 0.000000000000000000, 1.000000000000000000 ) ) ;
#6288=EDGE_CURVE ( 'NONE', #17511, #2792, #2654, .T. ) ;
#6291=AXIS2_PLACEMENT_3D ( 'NONE', #13878, #3315, #9272 ) ;
#6293=VECTOR ( 'NONE', #5427, 1000.000000000000000 ) ;
#6298=DIRECTION ( 'NONE',  ( -0.000000000000000000, -0.000000000000000000, -1.000000000000000000 ) ) ;
#6301=EDGE_CURVE ( 'NONE', #9525, #12297, #14387, .T. ) ;
#6306=CIRCLE ( 'NONE', #18547, 20.00000000000000000 ) ;
#6309=CARTESIAN_POINT ( 'NONE',  ( -9.037824375505568497, -2.158539001597504559, -9.000000000000000000 ) ) ;
#6319=VECTOR ( 'NONE', #5294, 1000.000000000000000 ) ;
#6328=VERTEX_POINT ( 'NONE', #4107 ) ;
#6329=EDGE_CURVE ( 'NONE', #660, #17716, #11443, .T. ) ;
#6332=EDGE_CURVE ( 'NONE', #10940, #8510, #4096, .T. ) ;
#6336=VERTEX_POINT ( 'NONE', #17449 ) ;
#6338=CARTESIAN_POINT ( 'NONE',  ( -12.54977455159113475, -35.57251292194792569, -9.000000000000000000 ) ) ;
#6342=CARTESIAN_POINT ( 'NONE',  ( 15.51323935927256237, -7.377028694403341191, 0.000000000000000000 ) ) ;
#6351=ORIENTED_EDGE ( 'NONE', *, *, #5063, .T. ) ;
#6355=EDGE_LOOP ( 'NONE', ( #1115, #564, #14181, #14168 ) ) ;
#6363=LINE ( 'NONE', #13990, #14093 ) ;
#6367=ORIENTED_EDGE ( 'NONE', *, *, #3057, .F. ) ;
#6368=ORIENTED_EDGE ( 'NONE', *, *, #11953, .F. ) ;
#6388=CIRCLE ( 'NONE', #17063, 20.00000000000000000 ) ;
#6393=EDGE_CURVE ( 'NONE', #7648, #7897, #4406, .T. ) ;
#6401=CARTESIAN_POINT ( 'NONE',  ( -3.158233816355195955, -0.4370479853238878887, -9.000000000000000000 ) ) ;
#6406=DIRECTION ( 'NONE',  ( 0.6691306063588571273, 0.7431448254773952433, 0.000000000000000000 ) ) ;
#6410=EDGE_CURVE ( 'NONE', #11107, #15438, #6273, .T. ) ;
#6413=ORIENTED_EDGE ( 'NONE', *, *, #5168, .F. ) ;
#6417=DIRECTION ( 'NONE',  ( -0.000000000000000000, -0.000000000000000000, -1.000000000000000000 ) ) ;
#6434=VERTEX_POINT ( 'NONE', #3028 ) ;
#6442=CIRCLE ( 'NONE', #8947, 0.9999999999999991118 ) ;
#6444=CARTESIAN_POINT ( 'NONE',  ( 15.51323935927283237, -32.62297130559633018, -9.000000000000000000 ) ) ;
#6446=DIRECTION ( 'NONE',  ( 1.000000000000000000, 0.000000000000000000, 0.000000000000000000 ) ) ;
#6456=ORIENTED_EDGE ( 'NONE', *, *, #3903, .T. ) ;
#6459=DIRECTION ( 'NONE',  ( -0.9135454576425982021, -0.4067366430758060925, 0.000000000000000000 ) ) ;
#6461=ORIENTED_EDGE ( 'NONE', *, *, #15006, .T. ) ;
#6465=VERTEX_POINT ( 'NONE', #16748 ) ;
#6466=CARTESIAN_POINT ( 'NONE',  ( -17.32050807568879236, -10.00000000000004263, -9.000000000000000000 ) ) ;
#6485=DIRECTION ( 'NONE',  ( 1.000000000000000000, 0.000000000000000000, 0.000000000000000000 ) ) ;
#6497=ADVANCED_FACE ( 'NONE', ( #13789 ), #18131, .F. ) ;
#6503=EDGE_CURVE ( 'NONE', #8420, #17731, #2560, .T. ) ;
#6513=VERTEX_POINT ( 'NONE', #555 ) ;
#6517=DIRECTION ( 'NONE',  ( 0.000000000000000000, -0.000000000000000000, 1.000000000000000000 ) ) ;
#6526=CARTESIAN_POINT ( 'NONE',  ( 7.211304515372446211, -1.345319965580511479, 0.000000000000000000 ) ) ;
#6535=ORIENTED_EDGE ( 'NONE', *, *, #6092, .F. ) ;
#6537=CARTESIAN_POINT ( 'NONE',  ( -11.75570504584937481, -36.18033988749900942, -9.000000000000000000 ) ) ;
#6538=VERTEX_POINT ( 'NONE', #13967 ) ;
#6554=CARTESIAN_POINT ( 'NONE',  ( -18.68843350152494054, -12.87662627267948956, 0.000000000000000000 ) ) ;
#6555=FILL_AREA_STYLE ('',( #17160 ) ) ;
#6564=EDGE_LOOP ( 'NONE', ( #8593, #13216, #15455, #16862 ) ) ;
#6565=EDGE_CURVE ( 'NONE', #6328, #16569, #9186, .T. ) ;
#6570=DIRECTION ( 'NONE',  ( -0.000000000000000000, -0.000000000000000000, 1.000000000000000000 ) ) ;
#6576=CIRCLE ( 'NONE', #18499, 20.00000000000000000 ) ;
#6580=VERTEX_POINT ( 'NONE', #15169 ) ;
#6584=AXIS2_PLACEMENT_3D ( 'NONE', #5174, #16772, #15383 ) ;
#6589=CARTESIAN_POINT ( 'NONE',  ( 5.000000000000003553, -20.00000000000000000, 9.000000000000000000 ) ) ;
#6606=CARTESIAN_POINT ( 'NONE',  ( 2.449293598294706513E-15, -20.00000000000000000, -9.000000000000000000 ) ) ;
#6633=EDGE_CURVE ( 'NONE', #17604, #13178, #7995, .T. ) ;
#6648=VECTOR ( 'NONE', #13279, 1000.000000000000000 ) ;
#6650=CARTESIAN_POINT ( 'NONE',  ( 7.211304515372821022, -38.65468003441933575, 9.000000000000000000 ) ) ;
#6652=DIRECTION ( 'NONE',  ( 0.000000000000000000, -0.000000000000000000, 1.000000000000000000 ) ) ;
#6657=CYLINDRICAL_SURFACE ( 'NONE', #15285, 20.00000000000000000 ) ;
#6663=CARTESIAN_POINT ( 'NONE',  ( -14.17539641854921229, -5.891203581560112923, 0.000000000000000000 ) ) ;
#6670=DIRECTION ( 'NONE',  ( -0.000000000000000000, -0.000000000000000000, -1.000000000000000000 ) ) ;
#6684=CARTESIAN_POINT ( 'NONE',  ( 2.449293598294706513E-15, -20.00000000000000000, 9.000000000000000000 ) ) ;
#6701=EDGE_LOOP ( 'NONE', ( #13366, #5549, #14200, #4093 ) ) ;
#6706=CARTESIAN_POINT ( 'NONE',  ( 2.449293598294706513E-15, -20.00000000000000000, -9.000000000000000000 ) ) ;
#6716=LINE ( 'NONE', #5247, #3687 ) ;
#6725=CARTESIAN_POINT ( 'NONE',  ( 11.75570504584960041, -36.18033988749885310, -9.000000000000000000 ) ) ;
#6734=ORIENTED_EDGE ( 'NONE', *, *, #11665, .T. ) ;
#6736=DIRECTION ( 'NONE',  ( -0.000000000000000000, 0.000000000000000000, 1.000000000000000000 ) ) ;
#6741=CARTESIAN_POINT ( 'NONE',  ( 19.97007065299861139, -18.90625500492856759, 0.000000000000000000 ) ) ;
#6749=EDGE_CURVE ( 'NONE', #9866, #1761, #1288, .T. ) ;
#6753=CARTESIAN_POINT ( 'NONE',  ( 2.449293598294706513E-15, -20.00000000000000000, -9.000000000000000000 ) ) ;
#6756=ORIENTED_EDGE ( 'NONE', *, *, #10945, .F. ) ;
#6780=AXIS2_PLACEMENT_3D ( 'NONE', #5027, #3470, #1998 ) ;
#6781=DIRECTION ( 'NONE',  ( -0.6691306063588624564, 0.7431448254773903583, 0.000000000000000000 ) ) ;
#6782=CARTESIAN_POINT ( 'NONE',  ( 2.449293598294706513E-15, -20.00000000000000000, -9.000000000000000000 ) ) ;
#6788=DIRECTION ( 'NONE',  ( -0.4999999999999933942, -0.8660254037844425934, 0.000000000000000000 ) ) ;
#6792=DIRECTION ( 'NONE',  ( 0.000000000000000000, 0.000000000000000000, 1.000000000000000000 ) ) ;
#6794=EDGE_LOOP ( 'NONE', ( #8575, #4159, #9475, #4346 ) ) ;
#6795=VERTEX_POINT ( 'NONE', #7207 ) ;
#6799=VERTEX_POINT ( 'NONE', #8963 ) ;
#6801=EDGE_LOOP ( 'NONE', ( #11716, #6756, #12178, #7577 ) ) ;
#6807=ORIENTED_EDGE ( 'NONE', *, *, #15756, .T. ) ;
#6808=CIRCLE ( 'NONE', #11176, 20.00000000000000000 ) ;
#6820=CARTESIAN_POINT ( 'NONE',  ( 5.130877905917027526, -0.6693483836014320065, 0.000000000000000000 ) ) ;
#6825=VECTOR ( 'NONE', #14, 1000.000000000000000 ) ;
#6827=CARTESIAN_POINT ( 'NONE',  ( -18.68843350152489080, -27.12337372732064011, 9.000000000000000000 ) ) ;
#6830=LINE ( 'NONE', #3995, #10825 ) ;
#6841=DIRECTION ( 'NONE',  ( -0.000000000000000000, -0.000000000000000000, 1.000000000000000000 ) ) ;
#6850=CIRCLE ( 'NONE', #11538, 1.000000000000000444 ) ;
#6851=EDGE_CURVE ( 'NONE', #18532, #16520, #1612, .T. ) ;
#6870=EDGE_CURVE ( 'NONE', #11790, #9875, #18226, .T. ) ;
#6873=CIRCLE ( 'NONE', #18803, 20.00000000000000000 ) ;
#6875=CYLINDRICAL_SURFACE ( 'NONE', #3363, 20.00000000000000000 ) ;
#6894=AXIS2_PLACEMENT_3D ( 'NONE', #7415, #13392, #10248 ) ;
#6904=CARTESIAN_POINT ( 'NONE',  ( -16.79901371501579632, -30.85325472854623285, -9.000000000000000000 ) ) ;
#6913=AXIS2_PLACEMENT_3D ( 'NONE', #5729, #2898, #9147 ) ;
#6917=AXIS2_PLACEMENT_3D ( 'NONE', #2483, #12756, #9603 ) ;
#6919=DIRECTION ( 'NONE',  ( 1.000000000000000000, 0.000000000000000000, 0.000000000000000000 ) ) ;
#6930=VERTEX_POINT ( 'NONE', #5640 ) ;
#6933=CARTESIAN_POINT ( 'NONE',  ( -8.134732861516020819, -1.729090847147989773, 9.000000000000000000 ) ) ;
#6947=VERTEX_POINT ( 'NONE', #4176 ) ;
#6949=PRESENTATION_STYLE_ASSIGNMENT (( #8411 ) ) ;
#6953=VERTEX_POINT ( 'NONE', #2724 ) ;
#6954=CARTESIAN_POINT ( 'NONE',  ( 14.17539641854901689, -5.891203581559916636, 0.000000000000000000 ) ) ;
#6984=ADVANCED_FACE ( 'NONE', ( #14648 ), #1234, .T. ) ;
#7004=DIRECTION ( 'NONE',  ( -4.082155997157844188E-16, 1.000000000000000000, 0.000000000000000000 ) ) ;
#7006=CIRCLE ( 'NONE', #10442, 5.000000000000000888 ) ;
#7029=DIRECTION ( 'NONE',  ( 1.000000000000000000, 0.000000000000000000, 0.000000000000000000 ) ) ;
#7034=LINE ( 'NONE', #677, #9532 ) ;
#7038=AXIS2_PLACEMENT_3D ( 'NONE', #14089, #14486, #8305 ) ;
#7074=CYLINDRICAL_SURFACE ( 'NONE', #18719, 1.000000000000000888 ) ;
#7088=ORIENTED_EDGE ( 'NONE', *, *, #11119, .T. ) ;
#7089=DIRECTION ( 'NONE',  ( -0.9781476007338065770, 0.2079116908177552348, 0.000000000000000000 ) ) ;
#7092=DIRECTION ( 'NONE',  ( 0.6691306063588571273, 0.7431448254773952433, 0.000000000000000000 ) ) ;
#7095=CARTESIAN_POINT ( 'NONE',  ( -18.89043790736545603, -22.09056926535314602, -9.000000000000000000 ) ) ;
#7108=ADVANCED_FACE ( 'NONE', ( #15431 ), #2009, .F. ) ;
#7113=ORIENTED_EDGE ( 'NONE', *, *, #17739, .T. ) ;
#7117=CARTESIAN_POINT ( 'NONE',  ( -1.000000000000000000, -14.00000000000000000, 8.999999999999998224 ) ) ;
#7130=FACE_OUTER_BOUND ( 'NONE', #13979, .T. ) ;
#7133=CARTESIAN_POINT ( 'NONE',  ( 2.449293598294706513E-15, -20.00000000000000000, -9.000000000000000000 ) ) ;
#7137=DIRECTION ( 'NONE',  ( 0.000000000000000000, -0.000000000000000000, 1.000000000000000000 ) ) ;
#7138=ADVANCED_FACE ( 'NONE', ( #18974 ), #8258, .F. ) ;
#7145=CARTESIAN_POINT ( 'NONE',  ( 3.175194142252359519, -39.74634503291702003, 0.000000000000000000 ) ) ;
#7150=DIRECTION ( 'NONE',  ( 0.000000000000000000, 0.000000000000000000, -1.000000000000000000 ) ) ;
#7154=CIRCLE ( 'NONE', #12162, 20.00000000000000000 ) ;
#7159=CARTESIAN_POINT ( 'NONE',  ( -14.86289650954790886, -6.617387872822862782, -9.000000000000000000 ) ) ;
#7165=CARTESIAN_POINT ( 'NONE',  ( 0.9996874511566150590, -39.97499999999999432, 9.000000000000000000 ) ) ;
#7169=ORIENTED_EDGE ( 'NONE', *, *, #8107, .T. ) ;
#7173=CARTESIAN_POINT ( 'NONE',  ( 19.30627432446641123, -14.77814480204120784, 9.000000000000000000 ) ) ;
#7178=AXIS2_PLACEMENT_3D ( 'NONE', #8467, #15729, #17112 ) ;
#7191=AXIS2_PLACEMENT_3D ( 'NONE', #18762, #15606, #9905 ) ;
#7207=CARTESIAN_POINT ( 'NONE',  ( -5.130877905917148318, -39.33065161639853358, -9.000000000000000000 ) ) ;
#7212=ORIENTED_EDGE ( 'NONE', *, *, #13223, .F. ) ;
#7218=DIRECTION ( 'NONE',  ( 0.8090169943749464521, 0.5877852522924744694, 0.000000000000000000 ) ) ;
#7232=EDGE_CURVE ( 'NONE', #17315, #8654, #13814, .T. ) ;
#7237=EDGE_CURVE ( 'NONE', #7750, #4148, #13188, .T. ) ;
#7245=ADVANCED_FACE ( 'NONE', ( #5514 ), #9822, .F. ) ;
#7249=CARTESIAN_POINT ( 'NONE',  ( -19.99999999999999645, -20.00000000000000000, 9.000000000000000000 ) ) ;
#7254=DIRECTION ( 'NONE',  ( 0.000000000000000000, 0.000000000000000000, 1.000000000000000000 ) ) ;
#7267=ADVANCED_FACE ( 'NONE', ( #16487 ), #6183, .T. ) ;
#7272=FACE_OUTER_BOUND ( 'NONE', #1323, .T. ) ;
#7274=CARTESIAN_POINT ( 'NONE',  ( 15.51323935927256237, -7.377028694403341191, 9.000000000000000000 ) ) ;
#7290=DIRECTION ( 'NONE',  ( 0.000000000000000000, 0.000000000000000000, 1.000000000000000000 ) ) ;
#7309=DIRECTION ( 'NONE',  ( -0.9135454576426043083, 0.4067366430757925477, 0.000000000000000000 ) ) ;
#7314=EDGE_LOOP ( 'NONE', ( #12545, #2817, #13298, #19309 ) ) ;
#7315=CYLINDRICAL_SURFACE ( 'NONE', #2046, 1.000000000000000000 ) ;
#7318=CARTESIAN_POINT ( 'NONE',  ( 2.449293598294706513E-15, -20.00000000000000000, 9.000000000000000000 ) ) ;
#7324=CIRCLE ( 'NONE', #13885, 0.9999999999999991118 ) ;
#7329=DIRECTION ( 'NONE',  ( -0.8090169943749430104, -0.5877852522924791323, 0.000000000000000000 ) ) ;
#7344=FACE_OUTER_BOUND ( 'NONE', #9471, .T. ) ;
#7347=AXIS2_PLACEMENT_3D ( 'NONE', #13810, #6266, #9485 ) ;
#7357=EDGE_CURVE ( 'NONE', #12063, #17098, #3041, .T. ) ;
#7368=CARTESIAN_POINT ( 'NONE',  ( -5.130877905917283321, -0.6693483836015015065, 0.000000000000000000 ) ) ;
#7378=DIRECTION ( 'NONE',  ( -0.6691306063588506881, -0.7431448254774009055, 0.000000000000000000 ) ) ;
#7386=DIRECTION ( 'NONE',  ( 0.000000000000000000, 0.000000000000000000, 1.000000000000000000 ) ) ;
#7395=DIRECTION ( 'NONE',  ( -9.858538378746663627E-23, 5.031452844637890958E-23, -1.000000000000000000 ) ) ;
#7397=CIRCLE ( 'NONE', #5831, 0.9999999999999980016 ) ;
#7406=ORIENTED_EDGE ( 'NONE', *, *, #12626, .T. ) ;
#7413=DIRECTION ( 'NONE',  ( 0.1045284632676494602, 0.9945218953682738450, 0.000000000000000000 ) ) ;
#7415=CARTESIAN_POINT ( 'NONE',  ( 0.000000000000000000, 0.000000000000000000, -9.000000000000000000 ) ) ;
#7419=ORIENTED_EDGE ( 'NONE', *, *, #12496, .F. ) ;
#7420=CARTESIAN_POINT ( 'NONE',  ( 2.449293598294706513E-15, -20.00000000000000000, 9.000000000000000000 ) ) ;
#7447=VECTOR ( 'NONE', #19148, 1000.000000000000000 ) ;
#7462=AXIS2_PLACEMENT_3D ( 'NONE', #17162, #9687, #5474 ) ;
#7464=LINE ( 'NONE', #7368, #1254 ) ;
#7469=DIRECTION ( 'NONE',  ( -0.000000000000000000, -0.000000000000000000, 1.000000000000000000 ) ) ;
#7479=ORIENTED_EDGE ( 'NONE', *, *, #2108, .F. ) ;
#7480=EDGE_CURVE ( 'NONE', #3535, #6538, #1807, .T. ) ;
#7483=ORIENTED_EDGE ( 'NONE', *, *, #18402, .T. ) ;
#7489=EDGE_CURVE ( 'NONE', #15388, #6930, #6168, .T. ) ;
#7490=CARTESIAN_POINT ( 'NONE',  ( 1.000000000000002442, -20.00000000000000000, 8.999999999999998224 ) ) ;
#7491=VERTEX_POINT ( 'NONE', #10716 ) ;
#7495=ADVANCED_FACE ( 'NONE', ( #10616 ), #3273, .F. ) ;
#7496=CARTESIAN_POINT ( 'NONE',  ( -19.89043790736547379, -17.90943073464699609, -9.000000000000000000 ) ) ;
#7501=CYLINDRICAL_SURFACE ( 'NONE', #5966, 20.00000000000000000 ) ;
#7504=CIRCLE ( 'NONE', #18475, 0.9999999999999991118 ) ;
#7511=VERTEX_POINT ( 'NONE', #8864 ) ;
#7512=DIRECTION ( 'NONE',  ( 1.000000000000000000, 0.000000000000000000, 0.000000000000000000 ) ) ;
#7535=CIRCLE ( 'NONE', #17558, 20.00000000000000000 ) ;
#7548=DIRECTION ( 'NONE',  ( 0.000000000000000000, 0.000000000000000000, 1.000000000000000000 ) ) ;
#7554=DIRECTION ( 'NONE',  ( -0.000000000000000000, 0.000000000000000000, 1.000000000000000000 ) ) ;
#7577=ORIENTED_EDGE ( 'NONE', *, *, #9501, .T. ) ;
#7580=CARTESIAN_POINT ( 'NONE',  ( -17.32050807568872841, -30.00000000000008171, -9.000000000000000000 ) ) ;
#7587=EDGE_CURVE ( 'NONE', #12063, #12327, #15516, .T. ) ;
#7604=CARTESIAN_POINT ( 'NONE',  ( -11.75570504584948139, -3.819660112501066518, 9.000000000000000000 ) ) ;
#7609=ORIENTED_EDGE ( 'NONE', *, *, #14897, .T. ) ;
#7621=LINE ( 'NONE', #18129, #2580 ) ;
#7636=EDGE_CURVE ( 'NONE', #10464, #16376, #17006, .T. ) ;
#7638=CARTESIAN_POINT ( 'NONE',  ( -19.76107906696389094, -23.08216711247160546, 9.000000000000000000 ) ) ;
#7644=CIRCLE ( 'NONE', #13591, 20.00000000000000000 ) ;
#7648=VERTEX_POINT ( 'NONE', #16908 ) ;
#7675=DIRECTION ( 'NONE',  ( 0.000000000000000000, 0.000000000000000000, 1.000000000000000000 ) ) ;
#7684=AXIS2_PLACEMENT_3D ( 'NONE', #7848, #9126, #16400 ) ;
#7688=VERTEX_POINT ( 'NONE', #3559 ) ;
#7695=CARTESIAN_POINT ( 'NONE',  ( 3.175194142251959395, -0.2536549670829221781, 9.000000000000000000 ) ) ;
#7701=ORIENTED_EDGE ( 'NONE', *, *, #13276, .F. ) ;
#7704=EDGE_CURVE ( 'NONE', #3574, #2792, #16504, .T. ) ;
#7707=AXIS2_PLACEMENT_3D ( 'NONE', #16183, #12054, #16577 ) ;
#7710=DIRECTION ( 'NONE',  ( -0.000000000000000000, 0.000000000000000000, 1.000000000000000000 ) ) ;
#7712=CARTESIAN_POINT ( 'NONE',  ( 11.75570504584926468, -3.819660112500910198, -9.000000000000000000 ) ) ;
#7713=ORIENTED_EDGE ( 'NONE', *, *, #7636, .F. ) ;
#7722=VERTEX_POINT ( 'NONE', #17754 ) ;
#7723=FACE_OUTER_BOUND ( 'NONE', #6794, .T. ) ;
#7725=EDGE_LOOP ( 'NONE', ( #8874, #10715, #3987, #5167 ) ) ;
#7727=ORIENTED_EDGE ( 'NONE', *, *, #10126, .T. ) ;
#7732=CARTESIAN_POINT ( 'NONE',  ( 19.89043790736549155, -22.09056926535286891, -9.000000000000000000 ) ) ;
#7743=AXIS2_PLACEMENT_3D ( 'NONE', #10010, #5607, #16014 ) ;
#7747=ORIENTED_EDGE ( 'NONE', *, *, #6221, .T. ) ;
#7749=PRODUCT_CONTEXT ( 'NONE', #17919, 'mechanical' ) ;
#7750=VERTEX_POINT ( 'NONE', #18871 ) ;
#7751=LINE ( 'NONE', #1880, #13313 ) ;
#7761=CARTESIAN_POINT ( 'NONE',  ( -16.79901371501580698, -30.85325472854621864, 0.000000000000000000 ) ) ;
#7768=CIRCLE ( 'NONE', #15268, 20.00000000000000000 ) ;
#7775=ORIENTED_EDGE ( 'NONE', *, *, #18888, .T. ) ;
#7777=VECTOR ( 'NONE', #14587, 1000.000000000000000 ) ;
#7781=DIRECTION ( 'NONE',  ( 0.5000000000000108802, -0.8660254037844323793, 0.000000000000000000 ) ) ;
#7808=CARTESIAN_POINT ( 'NONE',  ( -11.75570504584937481, -36.18033988749900942, 9.000000000000000000 ) ) ;
#7813=ORIENTED_EDGE ( 'NONE', *, *, #9310, .T. ) ;
#7816=CARTESIAN_POINT ( 'NONE',  ( -19.02113032590308705, -13.81966011250110249, -9.000000000000000000 ) ) ;
#7817=ORIENTED_EDGE ( 'NONE', *, *, #5434, .T. ) ;
#7818=DIRECTION ( 'NONE',  ( -1.000000000000000000, 0.000000000000000000, 0.000000000000000000 ) ) ;
#7830=ADVANCED_FACE ( 'NONE', ( #13427 ), #11952, .F. ) ;
#7838=AXIS2_PLACEMENT_3D ( 'NONE', #1057, #16155, #3902 ) ;
#7840=DIRECTION ( 'NONE',  ( -0.000000000000000000, -0.000000000000000000, -1.000000000000000000 ) ) ;
#7848=CARTESIAN_POINT ( 'NONE',  ( 19.89043790736544892, -17.90943073464672608, 9.000000000000000000 ) ) ;
#7852=CARTESIAN_POINT ( 'NONE',  ( 2.449293598294706513E-15, -20.00000000000000000, -9.000000000000000000 ) ) ;
#7855=DIRECTION ( 'NONE',  ( 0.000000000000000000, -0.000000000000000000, -1.000000000000000000 ) ) ;
#7894=ADVANCED_FACE ( 'NONE', ( #16864 ), #9292, .F. ) ;
#7897=VERTEX_POINT ( 'NONE', #7919 ) ;
#7904=DIRECTION ( 'NONE',  ( -0.000000000000000000, -0.000000000000000000, 1.000000000000000000 ) ) ;
#7907=DIRECTION ( 'NONE',  ( 1.000000000000000000, 0.000000000000000000, 0.000000000000000000 ) ) ;
#7912=ORIENTED_EDGE ( 'NONE', *, *, #7480, .F. ) ;
#7913=FACE_OUTER_BOUND ( 'NONE', #6094, .T. ) ;
#7919=CARTESIAN_POINT ( 'NONE',  ( 12.54977455159103705, -4.427487078051979275, -9.000000000000000000 ) ) ;
#7935=EDGE_CURVE ( 'NONE', #4800, #18559, #15184, .T. ) ;
#7942=CARTESIAN_POINT ( 'NONE',  ( 19.97007065299863271, -21.09374499507102740, 0.000000000000000000 ) ) ;
#7961=VERTEX_POINT ( 'NONE', #15097 ) ;
#7971=CARTESIAN_POINT ( 'NONE',  ( -4.158233816355195955, -0.4370479853238878887, -9.000000000000000000 ) ) ;
#7974=ORIENTED_EDGE ( 'NONE', *, *, #1677, .T. ) ;
#7995=LINE ( 'NONE', #6526, #9712 ) ;
#7999=CARTESIAN_POINT ( 'NONE',  ( 18.68843350152500093, -27.12337372732038432, 9.000000000000000000 ) ) ;
#8001=AXIS2_PLACEMENT_3D ( 'NONE', #15663, #1852, #668 ) ;
#8025=VECTOR ( 'NONE', #13848, 1000.000000000000000 ) ;
#8027=CARTESIAN_POINT ( 'NONE',  ( 17.32050807568866091, -9.999999999999797495, -9.000000000000000000 ) ) ;
#8030=CARTESIAN_POINT ( 'NONE',  ( -4.999999999999998224, -20.00000000000000000, 9.000000000000000000 ) ) ;
#8031=DIRECTION ( 'NONE',  ( 0.000000000000000000, 0.000000000000000000, 1.000000000000000000 ) ) ;
#8032=CARTESIAN_POINT ( 'NONE',  ( 2.449293598294706513E-15, -20.00000000000000000, -9.000000000000000000 ) ) ;
#8036=CYLINDRICAL_SURFACE ( 'NONE', #3155, 20.00000000000000000 ) ;
#8041=DIRECTION ( 'NONE',  ( 0.1045284632676635322, -0.9945218953682722907, 0.000000000000000000 ) ) ;
#8044=EDGE_LOOP ( 'NONE', ( #19305, #8387, #1216, #13473 ) ) ;
#8051=DIRECTION ( 'NONE',  ( 1.000000000000000000, 0.000000000000000000, 0.000000000000000000 ) ) ;
#8052=ORIENTED_EDGE ( 'NONE', *, *, #12618, .F. ) ;
#8058=FACE_OUTER_BOUND ( 'NONE', #18957, .T. ) ;
#8089=EDGE_CURVE ( 'NONE', #8295, #13819, #9778, .T. ) ;
#8093=AXIS2_PLACEMENT_3D ( 'NONE', #10758, #9375, #15367 ) ;
#8096=EDGE_LOOP ( 'NONE', ( #8198, #6119, #11453, #209 ) ) ;
#8102=CARTESIAN_POINT ( 'NONE',  ( -0.9999999999999995559, -15.10102051443364246, 15.00000000000000355 ) ) ;
#8103=ORIENTED_EDGE ( 'NONE', *, *, #2338, .T. ) ;
#8106=CIRCLE ( 'NONE', #8417, 1.000000000000000222 ) ;
#8107=EDGE_CURVE ( 'NONE', #10123, #5600, #17149, .T. ) ;
#8116=CARTESIAN_POINT ( 'NONE',  ( -11.75570504584937481, -36.18033988749900942, 9.000000000000000000 ) ) ;
#8118=ORIENTED_EDGE ( 'NONE', *, *, #1133, .F. ) ;
#8120=DIRECTION ( 'NONE',  ( -0.000000000000000000, -0.000000000000000000, 1.000000000000000000 ) ) ;
#8127=FACE_OUTER_BOUND ( 'NONE', #11014, .T. ) ;
#8133=DIRECTION ( 'NONE',  ( 1.000000000000000000, 0.000000000000000000, 0.000000000000000000 ) ) ;
#8136=LINE ( 'NONE', #12270, #14957 ) ;
#8139=LINE ( 'NONE', #597, #681 ) ;
#8140=CIRCLE ( 'NONE', #1290, 20.00000000000000000 ) ;
#8150=VECTOR ( 'NONE', #6841, 1000.000000000000000 ) ;
#8165=CARTESIAN_POINT ( 'NONE',  ( -17.32050807568879236, -10.00000000000004263, -9.000000000000000000 ) ) ;
#8167=FACE_OUTER_BOUND ( 'NONE', #7314, .T. ) ;
#8171=VERTEX_POINT ( 'NONE', #765 ) ;
#8176=CYLINDRICAL_SURFACE ( 'NONE', #13784, 20.00000000000000000 ) ;
#8179=ORIENTED_EDGE ( 'NONE', *, *, #4733, .T. ) ;
#8184=AXIS2_PLACEMENT_3D ( 'NONE', #4218, #8627, #8535 ) ;
#8192=ADVANCED_FACE ( 'NONE', ( #17350 ), #3909, .F. ) ;
#8194=EDGE_CURVE ( 'NONE', #7897, #8685, #14382, .T. ) ;
#8198=ORIENTED_EDGE ( 'NONE', *, *, #13469, .T. ) ;
#8200=ORIENTED_EDGE ( 'NONE', *, *, #4256, .T. ) ;
#8201=DIRECTION ( 'NONE',  ( -0.8090169943749430104, -0.5877852522924791323, 0.000000000000000000 ) ) ;
#8207=CARTESIAN_POINT ( 'NONE',  ( -7.134732861515892033, -38.27090915285207018, 9.000000000000000000 ) ) ;
#8217=CARTESIAN_POINT ( 'NONE',  ( -7.211304515372694901, -1.345319965580611843, -9.000000000000000000 ) ) ;
#8224=ORIENTED_EDGE ( 'NONE', *, *, #8499, .F. ) ;
#8231=DIRECTION ( 'NONE',  ( 1.000000000000000000, 0.000000000000000000, 0.000000000000000000 ) ) ;
#8235=CARTESIAN_POINT ( 'NONE',  ( -0.9996874511566102850, -0.02500000000000036915, 9.000000000000000000 ) ) ;
#8242=ORIENTED_EDGE ( 'NONE', *, *, #17259, .T. ) ;
#8247=AXIS2_PLACEMENT_3D ( 'NONE', #620, #2005, #13597 ) ;
#8248=CARTESIAN_POINT ( 'NONE',  ( 19.76107906696393357, -23.08216711247132835, -9.000000000000000000 ) ) ;
#8258=PLANE ( 'NONE',  #13503 ) ;
#8264=LINE ( 'NONE', #827, #15312 ) ;
#8268=DIRECTION ( 'NONE',  ( 0.000000000000000000, 0.000000000000000000, 1.000000000000000000 ) ) ;
#8271=CARTESIAN_POINT ( 'NONE',  ( -15.51323935927264586, -32.62297130559655045, 9.000000000000000000 ) ) ;
#8274=AXIS2_PLACEMENT_3D ( 'NONE', #8032, #317, #17079 ) ;
#8291=CIRCLE ( 'NONE', #11410, 1.000000000000000444 ) ;
#8293=CYLINDRICAL_SURFACE ( 'NONE', #12174, 20.00000000000000000 ) ;
#8295=VERTEX_POINT ( 'NONE', #10070 ) ;
#8299=ORIENTED_EDGE ( 'NONE', *, *, #14682, .F. ) ;
#8300=ADVANCED_FACE ( 'NONE', ( #11930 ), #11636, .T. ) ;
#8305=DIRECTION ( 'NONE',  ( -0.4999999999999933942, -0.8660254037844425934, 0.000000000000000000 ) ) ;
#8323=CIRCLE ( 'NONE', #16796, 1.000000000000000222 ) ;
#8328=FACE_OUTER_BOUND ( 'NONE', #10320, .T. ) ;
#8329=CIRCLE ( 'NONE', #7707, 1.000000000000000888 ) ;
#8337=VERTEX_POINT ( 'NONE', #5859 ) ;
#8338=CARTESIAN_POINT ( 'NONE',  ( 1.000000000000000444, -15.10102051443364246, 15.00000000000000355 ) ) ;
#8343=DIRECTION ( 'NONE',  ( 0.000000000000000000, 0.000000000000000000, 1.000000000000000000 ) ) ;
#8344=CARTESIAN_POINT ( 'NONE',  ( 5.000000000000003553, -20.00000000000000000, -8.999999999999998224 ) ) ;
#8347=AXIS2_PLACEMENT_3D ( 'NONE', #17957, #4515, #10474 ) ;
#8364=VERTEX_POINT ( 'NONE', #13874 ) ;
#8366=VERTEX_POINT ( 'NONE', #10545 ) ;
#8367=FACE_OUTER_BOUND ( 'NONE', #9448, .T. ) ;
#8371=ORIENTED_EDGE ( 'NONE', *, *, #1677, .F. ) ;
#8382=CARTESIAN_POINT ( 'NONE',  ( 2.449293598294706513E-15, -20.00000000000000000, 9.000000000000000000 ) ) ;
#8383=ORIENTED_EDGE ( 'NONE', *, *, #2638, .F. ) ;
#8387=ORIENTED_EDGE ( 'NONE', *, *, #1633, .F. ) ;
#8407=DIRECTION ( 'NONE',  ( 0.9781476007338055778, 0.2079116908177597867, 0.000000000000000000 ) ) ;
#8409=ORIENTED_EDGE ( 'NONE', *, *, #9328, .F. ) ;
#8411=SURFACE_STYLE_USAGE ( .BOTH. , #9685 ) ;
#8417=AXIS2_PLACEMENT_3D ( 'NONE', #12301, #250, #9253 ) ;
#8418=AXIS2_PLACEMENT_3D ( 'NONE', #11690, #2703, #8655 ) ;
#8420=VERTEX_POINT ( 'NONE', #3400 ) ;
#8429=CARTESIAN_POINT ( 'NONE',  ( 2.449293598294706513E-15, -20.00000000000000000, -9.000000000000000000 ) ) ;
#8436=AXIS2_PLACEMENT_3D ( 'NONE', #14733, #7386, #15198 ) ;
#8451=EDGE_LOOP ( 'NONE', ( #15084, #2250, #17992, #10025 ) ) ;
#8462=CARTESIAN_POINT ( 'NONE',  ( -8.134732861516020819, -1.729090847147989773, -9.000000000000000000 ) ) ;
#8465=CIRCLE ( 'NONE', #11903, 20.00000000000000000 ) ;
#8467=CARTESIAN_POINT ( 'NONE',  ( 2.449293598294706513E-15, -20.00000000000000000, 9.000000000000000000 ) ) ;
#8487=CIRCLE ( 'NONE', #10353, 20.00000000000000000 ) ;
#8499=EDGE_CURVE ( 'NONE', #3507, #15861, #14358, .T. ) ;
#8508=EDGE_CURVE ( 'NONE', #8366, #6538, #3365, .T. ) ;
#8510=VERTEX_POINT ( 'NONE', #2325 ) ;
#8529=FACE_OUTER_BOUND ( 'NONE', #8551, .T. ) ;
#8535=DIRECTION ( 'NONE',  ( 1.000000000000000000, 0.000000000000000000, 0.000000000000000000 ) ) ;
#8538=DIRECTION ( 'NONE',  ( 0.000000000000000000, -0.000000000000000000, -1.000000000000000000 ) ) ;
#8549=CARTESIAN_POINT ( 'NONE',  ( 2.449293598294706513E-15, -20.00000000000000000, 9.000000000000000000 ) ) ;
#8551=EDGE_LOOP ( 'NONE', ( #8299, #10752, #7727, #16318 ) ) ;
#8552=CYLINDRICAL_SURFACE ( 'NONE', #9824, 1.000000000000000888 ) ;
#8553=EDGE_CURVE ( 'NONE', #7688, #11251, #6716, .T. ) ;
#8575=ORIENTED_EDGE ( 'NONE', *, *, #1556, .F. ) ;
#8586=ORIENTED_EDGE ( 'NONE', *, *, #2312, .F. ) ;
#8593=ORIENTED_EDGE ( 'NONE', *, *, #9162, .F. ) ;
#8598=CARTESIAN_POINT ( 'NONE',  ( 17.79870116617255604, -29.12174527145369396, 0.000000000000000000 ) ) ;
#8607=CARTESIAN_POINT ( 'NONE',  ( -4.158233816355195955, -0.4370479853238878887, 9.000000000000000000 ) ) ;
#8608=AXIS2_PLACEMENT_3D ( 'NONE', #14797, #16576, #1374 ) ;
#8610=ORIENTED_EDGE ( 'NONE', *, *, #6870, .F. ) ;
#8614=CARTESIAN_POINT ( 'NONE',  ( -17.79870116617248499, -10.87825472854618170, 0.000000000000000000 ) ) ;
#8617=DIRECTION ( 'NONE',  ( -0.9135454576426043083, 0.4067366430757925477, 0.000000000000000000 ) ) ;
#8618=VERTEX_POINT ( 'NONE', #14464 ) ;
#8623=CARTESIAN_POINT ( 'NONE',  ( -8.134732861515892921, -38.27090915285207018, -9.000000000000000000 ) ) ;
#8624=CIRCLE ( 'NONE', #2699, 20.00000000000000000 ) ;
#8627=DIRECTION ( 'NONE',  ( -0.000000000000000000, -0.000000000000000000, 1.000000000000000000 ) ) ;
#8633=DIRECTION ( 'NONE',  ( -0.000000000000000000, -0.000000000000000000, 1.000000000000000000 ) ) ;
#8637=CIRCLE ( 'NONE', #3333, 1.000000000000000444 ) ;
#8638=CARTESIAN_POINT ( 'NONE',  ( -7.134732861515892033, -38.27090915285207018, -9.000000000000000000 ) ) ;
#8641=FACE_OUTER_BOUND ( 'NONE', #10654, .T. ) ;
#8654=VERTEX_POINT ( 'NONE', #8768 ) ;
#8655=DIRECTION ( 'NONE',  ( -1.000000000000000000, 0.000000000000000000, 0.000000000000000000 ) ) ;
#8671=DIRECTION ( 'NONE',  ( 0.000000000000000000, 0.000000000000000000, 1.000000000000000000 ) ) ;
#8674=DIRECTION ( 'NONE',  ( 1.000000000000000000, 0.000000000000000000, 0.000000000000000000 ) ) ;
#8685=VERTEX_POINT ( 'NONE', #18901 ) ;
#8694=DIRECTION ( 'NONE',  ( -0.000000000000000000, -0.000000000000000000, 1.000000000000000000 ) ) ;
#8697=EDGE_CURVE ( 'NONE', #1643, #1761, #5439, .T. ) ;
#8703=DIRECTION ( 'NONE',  ( 0.000000000000000000, 0.000000000000000000, 1.000000000000000000 ) ) ;
#8720=EDGE_CURVE ( 'NONE', #15947, #14101, #16856, .T. ) ;
#8723=DIRECTION ( 'NONE',  ( 0.1045284632676494602, 0.9945218953682738450, 0.000000000000000000 ) ) ;
#8737=CARTESIAN_POINT ( 'NONE',  ( 3.175194142251945184, -0.2536549670829196801, -9.000000000000000000 ) ) ;
#8738=EDGE_CURVE ( 'NONE', #15388, #18444, #6124, .T. ) ;
#8743=AXIS2_PLACEMENT_3D ( 'NONE', #6227, #16638, #12201 ) ;
#8751=CARTESIAN_POINT ( 'NONE',  ( -19.30627432446647518, -14.77814480204147785, -9.000000000000000000 ) ) ;
#8754=DIRECTION ( 'NONE',  ( 0.000000000000000000, 0.000000000000000000, 1.000000000000000000 ) ) ;
#8760=VERTEX_POINT ( 'NONE', #11999 ) ;
#8762=LINE ( 'NONE', #7490, #12733 ) ;
#8768=CARTESIAN_POINT ( 'NONE',  ( -16.79901371501587803, -9.146745271453902149, -9.000000000000000000 ) ) ;
#8774=AXIS2_PLACEMENT_3D ( 'NONE', #8116, #17153, #12433 ) ;
#8791=ORIENTED_EDGE ( 'NONE', *, *, #9510, .T. ) ;
#8793=CARTESIAN_POINT ( 'NONE',  ( 12.54977455159136568, -35.57251292194775516, -9.000000000000000000 ) ) ;
#8802=ADVANCED_FACE ( 'NONE', ( #10620 ), #1523, .T. ) ;
#8803=DIRECTION ( 'NONE',  ( 0.000000000000000000, 0.000000000000000000, 1.000000000000000000 ) ) ;
#8813=EDGE_CURVE ( 'NONE', #11790, #6465, #9241, .T. ) ;
#8816=DIRECTION ( 'NONE',  ( 0.3090169943749456194, 0.9510565162951541973, 0.000000000000000000 ) ) ;
#8825=CIRCLE ( 'NONE', #382, 1.000000000000001554 ) ;
#8832=ORIENTED_EDGE ( 'NONE', *, *, #12671, .F. ) ;
#8834=DIRECTION ( 'NONE',  ( 0.000000000000000000, 0.000000000000000000, 1.000000000000000000 ) ) ;
#8851=ADVANCED_FACE ( 'NONE', ( #18676 ), #16811, .T. ) ;
#8855=ORIENTED_EDGE ( 'NONE', *, *, #9867, .F. ) ;
#8857=VERTEX_POINT ( 'NONE', #6401 ) ;
#8861=ORIENTED_EDGE ( 'NONE', *, *, #14831, .F. ) ;
#8864=CARTESIAN_POINT ( 'NONE',  ( 3.175194142252359963, -39.74634503291702003, -9.000000000000000000 ) ) ;
#8865=CARTESIAN_POINT ( 'NONE',  ( 2.449293598294706513E-15, -20.00000000000000000, -9.000000000000000000 ) ) ;
#8873=ORIENTED_EDGE ( 'NONE', *, *, #7704, .F. ) ;
#8874=ORIENTED_EDGE ( 'NONE', *, *, #9965, .F. ) ;
#8903=ORIENTED_EDGE ( 'NONE', *, *, #7237, .F. ) ;
#8924=DIRECTION ( 'NONE',  ( 1.000000000000000000, 0.000000000000000000, 0.000000000000000000 ) ) ;
#8925=ADVANCED_FACE ( 'NONE', ( #11714 ), #7315, .F. ) ;
#8933=CIRCLE ( 'NONE', #3615, 20.00000000000000000 ) ;
#8936=LINE ( 'NONE', #10302, #18314 ) ;
#8937=FACE_OUTER_BOUND ( 'NONE', #15092, .T. ) ;
#8939=LINE ( 'NONE', #6104, #1703 ) ;
#8947=AXIS2_PLACEMENT_3D ( 'NONE', #18348, #11054, #12338 ) ;
#8950=CYLINDRICAL_SURFACE ( 'NONE', #9713, 5.000000000000000888 ) ;
#8963=CARTESIAN_POINT ( 'NONE',  ( 14.17539641854931176, -34.10879641843979471, 9.000000000000000000 ) ) ;
#8965=ORIENTED_EDGE ( 'NONE', *, *, #17186, .F. ) ;
#9040=VERTEX_POINT ( 'NONE', #14218 ) ;
#9053=DIRECTION ( 'NONE',  ( -1.000000000000000000, 0.000000000000000000, 0.000000000000000000 ) ) ;
#9060=CARTESIAN_POINT ( 'NONE',  ( -7.211304515372694901, -1.345319965580611843, 9.000000000000000000 ) ) ;
#9061=CIRCLE ( 'NONE', #17227, 20.00000000000000000 ) ;
#9073=EDGE_CURVE ( 'NONE', #15947, #18931, #16143, .T. ) ;
#9091=EDGE_CURVE ( 'NONE', #6947, #14650, #2386, .T. ) ;
#9096=VECTOR ( 'NONE', #17659, 1000.000000000000000 ) ;
#9097=EDGE_CURVE ( 'NONE', #3087, #4800, #16757, .T. ) ;
#9100=VECTOR ( 'NONE', #12248, 1000.000000000000000 ) ;
#9101=CIRCLE ( 'NONE', #3481, 1.000000000000000888 ) ;
#9103=DIRECTION ( 'NONE',  ( -1.000000000000000000, 0.000000000000000000, 0.000000000000000000 ) ) ;
#9107=ORIENTED_EDGE ( 'NONE', *, *, #15447, .F. ) ;
#9114=CARTESIAN_POINT ( 'NONE',  ( -19.89043790736547379, -17.90943073464699609, 9.000000000000000000 ) ) ;
#9126=DIRECTION ( 'NONE',  ( 0.000000000000000000, 0.000000000000000000, 1.000000000000000000 ) ) ;
#9132=CARTESIAN_POINT ( 'NONE',  ( 2.449293598294706513E-15, -20.00000000000000000, -9.000000000000000000 ) ) ;
#9138=ADVANCED_FACE ( 'NONE', ( #15903, #4041 ), #14813, .T. ) ;
#9147=DIRECTION ( 'NONE',  ( 1.000000000000000000, 0.000000000000000000, 0.000000000000000000 ) ) ;
#9160=EDGE_CURVE ( 'NONE', #18844, #3696, #4140, .T. ) ;
#9162=EDGE_CURVE ( 'NONE', #17604, #15949, #8933, .T. ) ;
#9173=ORIENTED_EDGE ( 'NONE', *, *, #17812, .F. ) ;
#9186=LINE ( 'NONE', #4963, #2863 ) ;
#9192=ORIENTED_EDGE ( 'NONE', *, *, #18396, .F. ) ;
#9197=EDGE_CURVE ( 'NONE', #6947, #12063, #183, .T. ) ;
#9201=CARTESIAN_POINT ( 'NONE',  ( 19.97007065299863271, -21.09374499507101319, -9.000000000000000000 ) ) ;
#9207=AXIS2_PLACEMENT_3D ( 'NONE', #721, #15426, #6788 ) ;
#9211=DIRECTION ( 'NONE',  ( -1.000000000000000000, 0.000000000000000000, 0.000000000000000000 ) ) ;
#9213=SHAPE_DEFINITION_REPRESENTATION ( #17125, #9916 ) ;
#9226=CARTESIAN_POINT ( 'NONE',  ( 4.158233816354936607, -0.4370479853238358192, 9.000000000000000000 ) ) ;
#9231=CARTESIAN_POINT ( 'NONE',  ( -14.17539641854910570, -34.10879641843999366, -9.000000000000000000 ) ) ;
#9237=DIRECTION ( 'NONE',  ( 1.000000000000000000, 0.000000000000000000, 0.000000000000000000 ) ) ;
#9241=LINE ( 'NONE', #18292, #12355 ) ;
#9248=ORIENTED_EDGE ( 'NONE', *, *, #9310, .F. ) ;
#9253=DIRECTION ( 'NONE',  ( 0.9135454576426006446, 0.4067366430758008189, 0.000000000000000000 ) ) ;
#9254=ORIENTED_EDGE ( 'NONE', *, *, #10706, .F. ) ;
#9260=CARTESIAN_POINT ( 'NONE',  ( 2.449293598294706513E-15, -20.00000000000000000, 9.000000000000000000 ) ) ;
#9272=DIRECTION ( 'NONE',  ( 1.000000000000000000, 0.000000000000000000, 0.000000000000000000 ) ) ;
#9276=EDGE_LOOP ( 'NONE', ( #19018, #5779, #4965, #14364 ) ) ;
#9292=CYLINDRICAL_SURFACE ( 'NONE', #1482, 1.000000000000000888 ) ;
#9302=DIRECTION ( 'NONE',  ( 0.000000000000000000, 0.000000000000000000, 1.000000000000000000 ) ) ;
#9307=DIRECTION ( 'NONE',  ( 0.1045284632676494602, 0.9945218953682738450, 0.000000000000000000 ) ) ;
#9309=DIRECTION ( 'NONE',  ( 0.9135454576426060846, -0.4067366430757887730, 0.000000000000000000 ) ) ;
#9310=EDGE_CURVE ( 'NONE', #16610, #12297, #1752, .T. ) ;
#9317=DIRECTION ( 'NONE',  ( 0.000000000000000000, 0.000000000000000000, 1.000000000000000000 ) ) ;
#9323=FACE_OUTER_BOUND ( 'NONE', #14121, .T. ) ;
#9328=EDGE_CURVE ( 'NONE', #17315, #18931, #7751, .T. ) ;
#9332=DIRECTION ( 'NONE',  ( 0.000000000000000000, 0.000000000000000000, 1.000000000000000000 ) ) ;
#9338=CARTESIAN_POINT ( 'NONE',  ( 15.51323935927282704, -32.62297130559633729, 9.000000000000000000 ) ) ;
#9349=AXIS2_PLACEMENT_3D ( 'NONE', #9735, #11106, #9635 ) ;
#9358=DIRECTION ( 'NONE',  ( 1.000000000000000000, 0.000000000000000000, 0.000000000000000000 ) ) ;
#9367=DIRECTION ( 'NONE',  ( 0.000000000000000000, -0.000000000000000000, -1.000000000000000000 ) ) ;
#9368=EDGE_CURVE ( 'NONE', #17098, #8171, #10587, .T. ) ;
#9370=EDGE_LOOP ( 'NONE', ( #2823, #15080, #11237, #1358 ) ) ;
#9373=EDGE_CURVE ( 'NONE', #2700, #5469, #11118, .T. ) ;
#9375=DIRECTION ( 'NONE',  ( -0.000000000000000000, -0.000000000000000000, 1.000000000000000000 ) ) ;
#9378=AXIS2_PLACEMENT_3D ( 'NONE', #10297, #11474, #17484 ) ;
#9379=EDGE_CURVE ( 'NONE', #12892, #6434, #15298, .T. ) ;
#9385=DIRECTION ( 'NONE',  ( 0.000000000000000000, -0.000000000000000000, 1.000000000000000000 ) ) ;
#9391=CARTESIAN_POINT ( 'NONE',  ( 12.54977455159135502, -35.57251292194776227, 0.000000000000000000 ) ) ;
#9407=CYLINDRICAL_SURFACE ( 'NONE', #13925, 20.00000000000000000 ) ;
#9411=CARTESIAN_POINT ( 'NONE',  ( 4.158233816354936607, -0.4370479853238358192, -9.000000000000000000 ) ) ;
#9432=CYLINDRICAL_SURFACE ( 'NONE', #17455, 1.000000000000000888 ) ;
#9433=ORIENTED_EDGE ( 'NONE', *, *, #18391, .F. ) ;
#9442=EDGE_CURVE ( 'NONE', #13074, #2657, #3001, .T. ) ;
#9447=VERTEX_POINT ( 'NONE', #17164 ) ;
#9448=EDGE_LOOP ( 'NONE', ( #96, #7701, #756, #14497 ) ) ;
#9469=ORIENTED_EDGE ( 'NONE', *, *, #13338, .F. ) ;
#9471=EDGE_LOOP ( 'NONE', ( #7479, #15874, #6734, #1443 ) ) ;
#9475=ORIENTED_EDGE ( 'NONE', *, *, #4076, .T. ) ;
#9482=UNCERTAINTY_MEASURE_WITH_UNIT (LENGTH_MEASURE( 1.000000000000000082E-05 ), #399, 'distance_accuracy_value', 'NONE');
#9485=DIRECTION ( 'NONE',  ( -0.1045284632676563297, 0.9945218953682731788, 0.000000000000000000 ) ) ;
#9491=CARTESIAN_POINT ( 'NONE',  ( 2.449293598294706513E-15, -20.00000000000000000, 9.000000000000000000 ) ) ;
#9493=ADVANCED_FACE ( 'NONE', ( #3536 ), #9407, .T. ) ;
#9497=ORIENTED_EDGE ( 'NONE', *, *, #2409, .F. ) ;
#9501=EDGE_CURVE ( 'NONE', #337, #9866, #1114, .T. ) ;
#9507=CARTESIAN_POINT ( 'NONE',  ( -9.037824375505429941, -37.84146099840256738, 9.000000000000000000 ) ) ;
#9510=EDGE_CURVE ( 'NONE', #11082, #4891, #8624, .T. ) ;
#9525=VERTEX_POINT ( 'NONE', #18450 ) ;
#9532=VECTOR ( 'NONE', #12725, 1000.000000000000000 ) ;
#9560=ORIENTED_EDGE ( 'NONE', *, *, #10126, .F. ) ;
#9586=ORIENTED_EDGE ( 'NONE', *, *, #8508, .T. ) ;
#9591=CLOSED_SHELL ( 'NONE', ( #5552, #10916, #12922, #5182, #1797, #1603, #14307, #3941, #17430, #12269, #5192, #18412, #8192, #3002, #7495, #7108, #3227, #9138, #15316, #18541, #8802, #8851, #11420, #12028, #17323, #13033, #13339, #9493, #14063, #16240, #12371, #10507, #7267, #9754, #4375, #6984, #4293, #16543, #9879, #13459, #5620, #8300, #17971, #10364, #10042, #13347, #4724, #14597, #3310, #19197, #11230, #8925, #17479, #6497, #10816, #16898, #11471, #15260, #7894, #10085, #15258, #7245, #3892, #7830, #18641, #5702, #1354, #4171, #3068, #13464, #10367, #3816, #4860, #930, #12121, #12136, #10727, #2827, #18808, #12488, #18299, #14530, #7138 ) ) ;
#9603=DIRECTION ( 'NONE',  ( 1.000000000000000000, 0.000000000000000000, 0.000000000000000000 ) ) ;
#9618=ORIENTED_EDGE ( 'NONE', *, *, #10945, .T. ) ;
#9619=CARTESIAN_POINT ( 'NONE',  ( 5.000000000000003553, -20.00000000000000000, 15.00000000000000355 ) ) ;
#9630=EDGE_CURVE ( 'NONE', #9875, #5600, #5815, .T. ) ;
#9632=EDGE_CURVE ( 'NONE', #1857, #17716, #8637, .T. ) ;
#9633=ORIENTED_EDGE ( 'NONE', *, *, #18347, .T. ) ;
#9635=DIRECTION ( 'NONE',  ( 4.082155997157843695E-16, -1.000000000000000000, 0.000000000000000000 ) ) ;
#9643=ORIENTED_EDGE ( 'NONE', *, *, #4413, .T. ) ;
#9650=CARTESIAN_POINT ( 'NONE',  ( -18.02113032590308705, -13.81966011250110249, -9.000000000000000000 ) ) ;
#9658=ORIENTED_EDGE ( 'NONE', *, *, #9162, .T. ) ;
#9670=AXIS2_PLACEMENT_3D ( 'NONE', #11715, #17822, #10151 ) ;
#9679=CARTESIAN_POINT ( 'NONE',  ( -19.02113032590304442, -26.18033988749903074, 9.000000000000000000 ) ) ;
#9684=DIRECTION ( 'NONE',  ( 1.000000000000000000, 0.000000000000000000, 0.000000000000000000 ) ) ;
#9685=SURFACE_SIDE_STYLE ('',( #777 ) ) ;
#9687=DIRECTION ( 'NONE',  ( 0.000000000000000000, 0.000000000000000000, 1.000000000000000000 ) ) ;
#9690=DIRECTION ( 'NONE',  ( 0.8090169943749464521, 0.5877852522924744694, 0.000000000000000000 ) ) ;
#9693=VERTEX_POINT ( 'NONE', #7249 ) ;
#9701=AXIS2_PLACEMENT_3D ( 'NONE', #2055, #11146, #15288 ) ;
#9712=VECTOR ( 'NONE', #12508, 1000.000000000000000 ) ;
#9713=AXIS2_PLACEMENT_3D ( 'NONE', #6026, #19191, #12087 ) ;
#9717=DIRECTION ( 'NONE',  ( -0.000000000000000000, -0.000000000000000000, -1.000000000000000000 ) ) ;
#9718=ORIENTED_EDGE ( 'NONE', *, *, #6027, .T. ) ;
#9719=DIRECTION ( 'NONE',  ( -0.9781476007338065770, 0.2079116908177552348, 0.000000000000000000 ) ) ;
#9721=EDGE_CURVE ( 'NONE', #14983, #12007, #10272, .T. ) ;
#9728=DIRECTION ( 'NONE',  ( 1.000000000000000000, 0.000000000000000000, 0.000000000000000000 ) ) ;
#9730=DIRECTION ( 'NONE',  ( 0.000000000000000000, 0.000000000000000000, 1.000000000000000000 ) ) ;
#9733=ORIENTED_EDGE ( 'NONE', *, *, #17186, .T. ) ;
#9735=CARTESIAN_POINT ( 'NONE',  ( -0.9999999999999976685, -20.00000000000000000, 8.999999999999998224 ) ) ;
#9741=CARTESIAN_POINT ( 'NONE',  ( 2.449293598294706513E-15, -20.00000000000000000, 9.000000000000000000 ) ) ;
#9745=ORIENTED_EDGE ( 'NONE', *, *, #6410, .F. ) ;
#9747=AXIS2_PLACEMENT_3D ( 'NONE', #17279, #12846, #18855 ) ;
#9754=ADVANCED_FACE ( 'NONE', ( #7723 ), #10664, .T. ) ;
#9755=DIRECTION ( 'NONE',  ( 0.000000000000000000, 0.000000000000000000, 1.000000000000000000 ) ) ;
#9760=CARTESIAN_POINT ( 'NONE',  ( -5.130877905917149207, -39.33065161639853358, 0.000000000000000000 ) ) ;
#9768=EDGE_CURVE ( 'NONE', #18532, #12297, #12710, .T. ) ;
#9778=LINE ( 'NONE', #571, #2755 ) ;
#9781=DIRECTION ( 'NONE',  ( -1.000000000000000000, 0.000000000000000000, 0.000000000000000000 ) ) ;
#9787=SHAPE_REPRESENTATION_RELATIONSHIP ( 'NONE' , 'NONE' ,  #9916, #11988 ) ;
#9791=EDGE_CURVE ( 'NONE', #6434, #7961, #198, .T. ) ;
#9803=DIRECTION ( 'NONE',  ( 0.000000000000000000, 0.000000000000000000, 1.000000000000000000 ) ) ;
#9807=DIRECTION ( 'NONE',  ( 0.000000000000000000, 0.000000000000000000, 1.000000000000000000 ) ) ;
#9822=CYLINDRICAL_SURFACE ( 'NONE', #16955, 1.000000000000000888 ) ;
#9823=DIRECTION ( 'NONE',  ( -1.000000000000000000, 0.000000000000000000, 0.000000000000000000 ) ) ;
#9824=AXIS2_PLACEMENT_3D ( 'NONE', #6195, #6101, #2883 ) ;
#9847=ORIENTED_EDGE ( 'NONE', *, *, #6288, .T. ) ;
#9849=ORIENTED_EDGE ( 'NONE', *, *, #3404, .T. ) ;
#9863=EDGE_CURVE ( 'NONE', #11041, #7511, #494, .T. ) ;
#9866=VERTEX_POINT ( 'NONE', #4408 ) ;
#9867=EDGE_CURVE ( 'NONE', #3997, #3999, #10376, .T. ) ;
#9868=EDGE_CURVE ( 'NONE', #3752, #11744, #1441, .T. ) ;
#9870=CARTESIAN_POINT ( 'NONE',  ( -11.75570504584937481, -36.18033988749900942, -9.000000000000000000 ) ) ;
#9873=CARTESIAN_POINT ( 'NONE',  ( 2.449293598294706513E-15, -20.00000000000000000, -9.000000000000000000 ) ) ;
#9874=AXIS2_PLACEMENT_3D ( 'NONE', #3139, #3234, #9103 ) ;
#9875=VERTEX_POINT ( 'NONE', #8207 ) ;
#9879=ADVANCED_FACE ( 'NONE', ( #469 ), #13800, .T. ) ;
#9888=CARTESIAN_POINT ( 'NONE',  ( -16.32050807568879236, -10.00000000000004263, -9.000000000000000000 ) ) ;
#9905=DIRECTION ( 'NONE',  ( -1.000000000000000000, 0.000000000000000000, 0.000000000000000000 ) ) ;
#9909=DIRECTION ( 'NONE',  ( 0.000000000000000000, 0.000000000000000000, 1.000000000000000000 ) ) ;
#9916=SHAPE_REPRESENTATION ( 'driver roller', ( #10359 ), #14982 ) ;
#9936=VECTOR ( 'NONE', #6570, 1000.000000000000000 ) ;
#9938=DIRECTION ( 'NONE',  ( -1.000000000000000000, 0.000000000000000000, 0.000000000000000000 ) ) ;
#9939=CIRCLE ( 'NONE', #10879, 20.00000000000000000 ) ;
#9942=DIRECTION ( 'NONE',  ( 0.000000000000000000, 0.000000000000000000, 1.000000000000000000 ) ) ;
#9951=AXIS2_PLACEMENT_3D ( 'NONE', #17360, #11945, #17845 ) ;
#9956=ORIENTED_EDGE ( 'NONE', *, *, #6215, .T. ) ;
#9957=DIRECTION ( 'NONE',  ( 0.000000000000000000, -0.000000000000000000, 1.000000000000000000 ) ) ;
#9965=EDGE_CURVE ( 'NONE', #13867, #2874, #3320, .T. ) ;
#9984=EDGE_LOOP ( 'NONE', ( #14265, #2343, #16540, #11598 ) ) ;
#9998=AXIS2_PLACEMENT_3D ( 'NONE', #14532, #8754, #17790 ) ;
#10000=LINE ( 'NONE', #12945, #4315 ) ;
#10003=AXIS2_PLACEMENT_3D ( 'NONE', #3189, #7675, #10712 ) ;
#10010=CARTESIAN_POINT ( 'NONE',  ( 2.449293598294706513E-15, -20.00000000000000000, 9.000000000000000000 ) ) ;
#10012=CIRCLE ( 'NONE', #14084, 20.00000000000000000 ) ;
#10024=VECTOR ( 'NONE', #12552, 1000.000000000000000 ) ;
#10025=ORIENTED_EDGE ( 'NONE', *, *, #8194, .F. ) ;
#10028=DIRECTION ( 'NONE',  ( 1.000000000000000000, 0.000000000000000000, 0.000000000000000000 ) ) ;
#10031=CIRCLE ( 'NONE', #1278, 1.000000000000000222 ) ;
#10042=ADVANCED_FACE ( 'NONE', ( #7913 ), #2346, .T. ) ;
#10047=AXIS2_PLACEMENT_3D ( 'NONE', #1526, #5743, #16531 ) ;
#10052=ORIENTED_EDGE ( 'NONE', *, *, #11665, .F. ) ;
#10059=ORIENTED_EDGE ( 'NONE', *, *, #18347, .F. ) ;
#10070=CARTESIAN_POINT ( 'NONE',  ( 18.68843350152500093, -27.12337372732038432, -9.000000000000000000 ) ) ;
#10074=DIRECTION ( 'NONE',  ( -0.3090169943749528914, 0.9510565162951518658, 0.000000000000000000 ) ) ;
#10079=CYLINDRICAL_SURFACE ( 'NONE', #17182, 0.9999999999999991118 ) ;
#10085=ADVANCED_FACE ( 'NONE', ( #5753 ), #18917, .F. ) ;
#10090=DIRECTION ( 'NONE',  ( -0.000000000000000000, -0.000000000000000000, -1.000000000000000000 ) ) ;
#10093=DIRECTION ( 'NONE',  ( -0.000000000000000000, -0.000000000000000000, -1.000000000000000000 ) ) ;
#10106=CARTESIAN_POINT ( 'NONE',  ( -15.51323935927273645, -7.377028694403556131, 0.000000000000000000 ) ) ;
#10117=CYLINDRICAL_SURFACE ( 'NONE', #132, 1.000000000000000888 ) ;
#10123=VERTEX_POINT ( 'NONE', #1150 ) ;
#10126=EDGE_CURVE ( 'NONE', #2700, #5077, #5551, .T. ) ;
#10128=ORIENTED_EDGE ( 'NONE', *, *, #2609, .T. ) ;
#10129=CARTESIAN_POINT ( 'NONE',  ( 2.449293598294706513E-15, -20.00000000000000000, 9.000000000000000000 ) ) ;
#10130=ORIENTED_EDGE ( 'NONE', *, *, #8738, .T. ) ;
#10138=CARTESIAN_POINT ( 'NONE',  ( 2.449293598294706513E-15, -20.00000000000000000, 9.000000000000000000 ) ) ;
#10143=CARTESIAN_POINT ( 'NONE',  ( -14.86289650954781649, -33.38261212717723936, -9.000000000000000000 ) ) ;
#10145=EDGE_CURVE ( 'NONE', #9447, #11744, #6830, .T. ) ;
#10149=EDGE_CURVE ( 'NONE', #666, #9447, #7397, .T. ) ;
#10151=DIRECTION ( 'NONE',  ( 1.000000000000000000, 0.000000000000000000, 0.000000000000000000 ) ) ;
#10157=ORIENTED_EDGE ( 'NONE', *, *, #17679, .T. ) ;
#10159=ORIENTED_EDGE ( 'NONE', *, *, #14534, .T. ) ;
#10164=DIRECTION ( 'NONE',  ( 0.8090169943749464521, 0.5877852522924744694, 0.000000000000000000 ) ) ;
#10190=CARTESIAN_POINT ( 'NONE',  ( 2.449293598294706513E-15, -20.00000000000000000, -9.000000000000000000 ) ) ;
#10194=AXIS2_PLACEMENT_3D ( 'NONE', #5580, #16275, #8617 ) ;
#10197=CIRCLE ( 'NONE', #1772, 1.000000000000000444 ) ;
#10198=CARTESIAN_POINT ( 'NONE',  ( -16.79901371501587803, -9.146745271453902149, 0.000000000000000000 ) ) ;
#10199=CARTESIAN_POINT ( 'NONE',  ( 14.86289650954772590, -6.617387872822656725, 9.000000000000000000 ) ) ;
#10206=EDGE_CURVE ( 'NONE', #14027, #8364, #8323, .T. ) ;
#10210=ORIENTED_EDGE ( 'NONE', *, *, #11285, .F. ) ;
#10213=CARTESIAN_POINT ( 'NONE',  ( 1.000000000000000444, -15.10102051443364246, -8.999999999999998224 ) ) ;
#10215=EDGE_CURVE ( 'NONE', #6434, #7511, #16308, .T. ) ;
#10223=EDGE_LOOP ( 'NONE', ( #2547, #7713, #3084, #14366 ) ) ;
#10240=ORIENTED_EDGE ( 'NONE', *, *, #10206, .F. ) ;
#10248=DIRECTION ( 'NONE',  ( 1.000000000000000000, 0.000000000000000000, 0.000000000000000000 ) ) ;
#10253=ORIENTED_EDGE ( 'NONE', *, *, #15623, .F. ) ;
#10262=AXIS2_PLACEMENT_3D ( 'NONE', #11005, #15330, #2299 ) ;
#10272=LINE ( 'NONE', #6954, #1766 ) ;
#10277=AXIS2_PLACEMENT_3D ( 'NONE', #1774, #11060, #2060 ) ;
#10292=AXIS2_PLACEMENT_3D ( 'NONE', #13388, #1438, #7413 ) ;
#10296=CARTESIAN_POINT ( 'NONE',  ( 2.449293598294706513E-15, -20.00000000000000000, 9.000000000000000000 ) ) ;
#10297=CARTESIAN_POINT ( 'NONE',  ( 2.449293598294706513E-15, -20.00000000000000000, 9.000000000000000000 ) ) ;
#10299=FACE_OUTER_BOUND ( 'NONE', #2319, .T. ) ;
#10302=CARTESIAN_POINT ( 'NONE',  ( 10.93224627749287592, -3.252283996668583033, 0.000000000000000000 ) ) ;
#10303=CIRCLE ( 'NONE', #7178, 20.00000000000000000 ) ;
#10313=ORIENTED_EDGE ( 'NONE', *, *, #10396, .F. ) ;
#10317=ORIENTED_EDGE ( 'NONE', *, *, #2312, .T. ) ;
#10320=EDGE_LOOP ( 'NONE', ( #14154, #8103, #16321, #5623 ) ) ;
#10325=DIRECTION ( 'NONE',  ( 0.000000000000000000, 0.000000000000000000, 1.000000000000000000 ) ) ;
#10333=AXIS2_PLACEMENT_3D ( 'NONE', #8607, #2452, #12925 ) ;
#10335=DIRECTION ( 'NONE',  ( -0.000000000000000000, 0.000000000000000000, 1.000000000000000000 ) ) ;
#10353=AXIS2_PLACEMENT_3D ( 'NONE', #9741, #16033, #2617 ) ;
#10354=ORIENTED_EDGE ( 'NONE', *, *, #9791, .T. ) ;
#10355=AXIS2_PLACEMENT_3D ( 'NONE', #3004, #16338, #7309 ) ;
#10359=AXIS2_PLACEMENT_3D ( 'NONE', #2871, #8834, #16191 ) ;
#10364=ADVANCED_FACE ( 'NONE', ( #3115 ), #2824, .T. ) ;
#10367=ADVANCED_FACE ( 'NONE', ( #13294 ), #4678, .F. ) ;
#10376=LINE ( 'NONE', #8102, #16479 ) ;
#10377=ORIENTED_EDGE ( 'NONE', *, *, #16491, .T. ) ;
#10383=CARTESIAN_POINT ( 'NONE',  ( 19.02113032590300890, -13.81966011250085025, -9.000000000000000000 ) ) ;
#10396=EDGE_CURVE ( 'NONE', #3609, #7688, #14719, .T. ) ;
#10404=CYLINDRICAL_SURFACE ( 'NONE', #19261, 1.000000000000000888 ) ;
#10425=CARTESIAN_POINT ( 'NONE',  ( -16.32050807568872841, -30.00000000000008171, -9.000000000000000000 ) ) ;
#10438=DIRECTION ( 'NONE',  ( -0.000000000000000000, 0.000000000000000000, 1.000000000000000000 ) ) ;
#10439=ORIENTED_EDGE ( 'NONE', *, *, #5807, .T. ) ;
#10442=AXIS2_PLACEMENT_3D ( 'NONE', #11996, #49, #13660 ) ;
#10450=CARTESIAN_POINT ( 'NONE',  ( -10.75570504584937304, -36.18033988749900942, 9.000000000000000000 ) ) ;
#10457=ORIENTED_EDGE ( 'NONE', *, *, #9373, .T. ) ;
#10461=AXIS2_PLACEMENT_3D ( 'NONE', #8623, #3732, #8231 ) ;
#10462=EDGE_CURVE ( 'NONE', #7491, #18559, #15357, .T. ) ;
#10464=VERTEX_POINT ( 'NONE', #7695 ) ;
#10474=DIRECTION ( 'NONE',  ( 1.000000000000000000, 0.000000000000000000, 0.000000000000000000 ) ) ;
#10475=AXIS2_PLACEMENT_3D ( 'NONE', #4124, #10093, #2671 ) ;
#10481=EDGE_CURVE ( 'NONE', #7648, #3535, #10012, .T. ) ;
#10485=EDGE_CURVE ( 'NONE', #14568, #6799, #7535, .T. ) ;
#10486=ORIENTED_EDGE ( 'NONE', *, *, #1871, .T. ) ;
#10504=CARTESIAN_POINT ( 'NONE',  ( -12.54977455159124133, -4.427487078052150693, 9.000000000000000000 ) ) ;
#10507=ADVANCED_FACE ( 'NONE', ( #634 ), #8176, .T. ) ;
#10514=ORIENTED_EDGE ( 'NONE', *, *, #10145, .T. ) ;
#10521=CARTESIAN_POINT ( 'NONE',  ( -4.158233816355060064, -39.56295201467614220, 9.000000000000000000 ) ) ;
#10522=DIRECTION ( 'NONE',  ( -0.000000000000000000, 0.000000000000000000, -1.000000000000000000 ) ) ;
#10532=CARTESIAN_POINT ( 'NONE',  ( 14.17539641854930998, -34.10879641843979471, 0.000000000000000000 ) ) ;
#10533=ORIENTED_EDGE ( 'NONE', *, *, #19242, .F. ) ;
#10541=DIRECTION ( 'NONE',  ( 1.000000000000000000, 0.000000000000000000, 0.000000000000000000 ) ) ;
#10545=CARTESIAN_POINT ( 'NONE',  ( 10.93224627749287592, -3.252283996668583477, 9.000000000000000000 ) ) ;
#10568=DIRECTION ( 'NONE',  ( -0.000000000000000000, 0.000000000000000000, 1.000000000000000000 ) ) ;
#10572=FACE_OUTER_BOUND ( 'NONE', #94, .T. ) ;
#10578=CARTESIAN_POINT ( 'NONE',  ( 16.79901371501595975, -30.85325472854598416, 0.000000000000000000 ) ) ;
#10581=ORIENTED_EDGE ( 'NONE', *, *, #14043, .F. ) ;
#10582=CYLINDRICAL_SURFACE ( 'NONE', #4646, 20.00000000000000000 ) ;
#10587=LINE ( 'NONE', #13728, #18035 ) ;
#10605=CIRCLE ( 'NONE', #1533, 0.9999999999999982236 ) ;
#10610=FACE_OUTER_BOUND ( 'NONE', #19159, .T. ) ;
#10615=ORIENTED_EDGE ( 'NONE', *, *, #2638, .T. ) ;
#10616=FACE_OUTER_BOUND ( 'NONE', #18312, .T. ) ;
#10617=CARTESIAN_POINT ( 'NONE',  ( 2.449293598294706513E-15, -20.00000000000000000, -9.000000000000000000 ) ) ;
#10620=FACE_OUTER_BOUND ( 'NONE', #6355, .T. ) ;
#10629=VERTEX_POINT ( 'NONE', #538 ) ;
#10633=DIRECTION ( 'NONE',  ( 1.000000000000000000, 0.000000000000000000, 0.000000000000000000 ) ) ;
#10637=DIRECTION ( 'NONE',  ( 0.000000000000000000, -0.000000000000000000, 1.000000000000000000 ) ) ;
#10641=CARTESIAN_POINT ( 'NONE',  ( -19.76107906696391225, -16.91783288752853665, -9.000000000000000000 ) ) ;
#10654=EDGE_LOOP ( 'NONE', ( #16617, #12620, #2984, #7483 ) ) ;
#10657=DIRECTION ( 'NONE',  ( 0.000000000000000000, 0.000000000000000000, 1.000000000000000000 ) ) ;
#10664=CYLINDRICAL_SURFACE ( 'NONE', #5500, 20.00000000000000000 ) ;
#10668=ORIENTED_EDGE ( 'NONE', *, *, #5822, .F. ) ;
#10676=CARTESIAN_POINT ( 'NONE',  ( -19.30627432446643610, -25.22185519795866782, -9.000000000000000000 ) ) ;
#10681=ORIENTED_EDGE ( 'NONE', *, *, #3423, .F. ) ;
#10682=DIRECTION ( 'NONE',  ( 1.000000000000000000, 0.000000000000000000, 0.000000000000000000 ) ) ;
#10684=EDGE_CURVE ( 'NONE', #2700, #9693, #8140, .T. ) ;
#10698=EDGE_CURVE ( 'NONE', #3553, #3573, #5340, .T. ) ;
#10705=EDGE_CURVE ( 'NONE', #18844, #16440, #9101, .T. ) ;
#10706=EDGE_CURVE ( 'NONE', #6580, #5943, #1610, .T. ) ;
#10712=DIRECTION ( 'NONE',  ( -0.5000000000000041078, 0.8660254037844362651, 0.000000000000000000 ) ) ;
#10715=ORIENTED_EDGE ( 'NONE', *, *, #2938, .T. ) ;
#10716=CARTESIAN_POINT ( 'NONE',  ( -5.130877905917283321, -0.6693483836015013955, 9.000000000000000000 ) ) ;
#10726=ORIENTED_EDGE ( 'NONE', *, *, #13125, .T. ) ;
#10727=ADVANCED_FACE ( 'NONE', ( #8367 ), #14345, .F. ) ;
#10740=DIRECTION ( 'NONE',  ( 0.000000000000000000, -0.000000000000000000, 1.000000000000000000 ) ) ;
#10752=ORIENTED_EDGE ( 'NONE', *, *, #10684, .F. ) ;
#10758=CARTESIAN_POINT ( 'NONE',  ( 19.89043790736544892, -17.90943073464672608, -9.000000000000000000 ) ) ;
#10760=DIRECTION ( 'NONE',  ( -0.9781476007338035794, -0.2079116908177690293, 0.000000000000000000 ) ) ;
#10764=CARTESIAN_POINT ( 'NONE',  ( 7.211304515372446211, -1.345319965580511479, 9.000000000000000000 ) ) ;
#10776=CYLINDRICAL_SURFACE ( 'NONE', #17497, 20.00000000000000000 ) ;
#10800=DIRECTION ( 'NONE',  ( -0.000000000000000000, -0.000000000000000000, 1.000000000000000000 ) ) ;
#10803=CARTESIAN_POINT ( 'NONE',  ( -3.175194142252083296, -39.74634503291706267, 9.000000000000000000 ) ) ;
#10804=EDGE_CURVE ( 'NONE', #3235, #6953, #8487, .T. ) ;
#10816=ADVANCED_FACE ( 'NONE', ( #1513 ), #17797, .F. ) ;
#10820=EDGE_LOOP ( 'NONE', ( #15924, #7817, #12342, #10514 ) ) ;
#10825=VECTOR ( 'NONE', #9957, 1000.000000000000000 ) ;
#10831=FACE_OUTER_BOUND ( 'NONE', #5333, .T. ) ;
#10835=CIRCLE ( 'NONE', #6146, 20.00000000000000000 ) ;
#10850=AXIS2_PLACEMENT_3D ( 'NONE', #13657, #12185, #2900 ) ;
#10851=ORIENTED_EDGE ( 'NONE', *, *, #10481, .F. ) ;
#10855=CARTESIAN_POINT ( 'NONE',  ( 2.449293598294706513E-15, -20.00000000000000000, -9.000000000000000000 ) ) ;
#10866=ORIENTED_EDGE ( 'NONE', *, *, #18396, .T. ) ;
#10875=EDGE_CURVE ( 'NONE', #9693, #15486, #4731, .T. ) ;
#10879=AXIS2_PLACEMENT_3D ( 'NONE', #14212, #9803, #18858 ) ;
#10881=DIRECTION ( 'NONE',  ( 0.9135454576426006446, 0.4067366430758008189, 0.000000000000000000 ) ) ;
#10889=DIRECTION ( 'NONE',  ( 1.000000000000000000, 0.000000000000000000, 0.000000000000000000 ) ) ;
#10890=AXIS2_PLACEMENT_3D ( 'NONE', #3918, #13516, #5870 ) ;
#10916=ADVANCED_FACE ( 'NONE', ( #10610 ), #8950, .F. ) ;
#10919=EDGE_LOOP ( 'NONE', ( #10059, #13771, #4972, #9469 ) ) ;
#10940=VERTEX_POINT ( 'NONE', #11887 ) ;
#10945=EDGE_CURVE ( 'NONE', #11695, #3362, #15681, .T. ) ;
#10946=DIRECTION ( 'NONE',  ( 0.3090169943749456194, 0.9510565162951541973, 0.000000000000000000 ) ) ;
#10947=VERTEX_POINT ( 'NONE', #18091 ) ;
#10948=DIRECTION ( 'NONE',  ( -0.000000000000000000, -0.000000000000000000, -1.000000000000000000 ) ) ;
#10952=ORIENTED_EDGE ( 'NONE', *, *, #9721, .F. ) ;
#10962=LINE ( 'NONE', #9391, #9100 ) ;
#10972=AXIS2_PLACEMENT_3D ( 'NONE', #18082, #18276, #12277 ) ;
#10975=CARTESIAN_POINT ( 'NONE',  ( -12.54977455159124133, -4.427487078052150693, 0.000000000000000000 ) ) ;
#10982=AXIS2_PLACEMENT_3D ( 'NONE', #7971, #526, #15141 ) ;
#11005=CARTESIAN_POINT ( 'NONE',  ( -19.02113032590308705, -13.81966011250110249, 9.000000000000000000 ) ) ;
#11010=CIRCLE ( 'NONE', #5070, 20.00000000000000000 ) ;
#11013=EDGE_LOOP ( 'NONE', ( #5581, #2269, #19289, #13765, #13745, #19404 ) ) ;
#11014=EDGE_LOOP ( 'NONE', ( #14911, #11717, #16583, #18687 ) ) ;
#11026=DIRECTION ( 'NONE',  ( 0.000000000000000000, 0.000000000000000000, 1.000000000000000000 ) ) ;
#11028=CARTESIAN_POINT ( 'NONE',  ( -13.86289650954781649, -33.38261212717723936, -9.000000000000000000 ) ) ;
#11035=PRODUCT_DEFINITION_FORMATION_WITH_SPECIFIED_SOURCE ( 'ANY', '', #11800, .NOT_KNOWN. ) ;
#11041=VERTEX_POINT ( 'NONE', #11086 ) ;
#11054=DIRECTION ( 'NONE',  ( 0.000000000000000000, 0.000000000000000000, 1.000000000000000000 ) ) ;
#11060=DIRECTION ( 'NONE',  ( 0.000000000000000000, 0.000000000000000000, 1.000000000000000000 ) ) ;
#11066=CARTESIAN_POINT ( 'NONE',  ( 2.449293598294706513E-15, -20.00000000000000000, 9.000000000000000000 ) ) ;
#11073=DIRECTION ( 'NONE',  ( -0.000000000000000000, -0.000000000000000000, 1.000000000000000000 ) ) ;
#11082=VERTEX_POINT ( 'NONE', #6444 ) ;
#11086=CARTESIAN_POINT ( 'NONE',  ( 5.130877905917432535, -39.33065161639846252, -9.000000000000000000 ) ) ;
#11104=ORIENTED_EDGE ( 'NONE', *, *, #12318, .F. ) ;
#11106=DIRECTION ( 'NONE',  ( -1.000000000000000000, -4.082155997157843695E-16, 0.000000000000000000 ) ) ;
#11107=VERTEX_POINT ( 'NONE', #761 ) ;
#11118=CIRCLE ( 'NONE', #1429, 1.000000000000000444 ) ;
#11119=EDGE_CURVE ( 'NONE', #12796, #2842, #5671, .T. ) ;
#11136=CARTESIAN_POINT ( 'NONE',  ( 2.449293598294706513E-15, -20.00000000000000000, 9.000000000000000000 ) ) ;
#11140=VERTEX_POINT ( 'NONE', #567 ) ;
#11146=DIRECTION ( 'NONE',  ( 0.000000000000000000, 0.000000000000000000, 1.000000000000000000 ) ) ;
#11152=CIRCLE ( 'NONE', #6780, 1.000000000000000000 ) ;
#11158=DIRECTION ( 'NONE',  ( -0.000000000000000000, -0.000000000000000000, 1.000000000000000000 ) ) ;
#11160=CIRCLE ( 'NONE', #1798, 1.000000000000000222 ) ;
#11161=LINE ( 'NONE', #18457, #10024 ) ;
#11163=CYLINDRICAL_SURFACE ( 'NONE', #10461, 1.000000000000000000 ) ;
#11168=AXIS2_PLACEMENT_3D ( 'NONE', #16702, #17645, #16068 ) ;
#11176=AXIS2_PLACEMENT_3D ( 'NONE', #13640, #18177, #6196 ) ;
#11184=CARTESIAN_POINT ( 'NONE',  ( -14.86289650954781649, -33.38261212717723936, 9.000000000000000000 ) ) ;
#11186=VERTEX_POINT ( 'NONE', #8793 ) ;
#11194=CIRCLE ( 'NONE', #17167, 1.000000000000000222 ) ;
#11200=CARTESIAN_POINT ( 'NONE',  ( 4.898587196589413026E-15, -40.00000000000000000, 9.000000000000000000 ) ) ;
#11207=DIRECTION ( 'NONE',  ( -1.000000000000000000, 0.000000000000000000, 0.000000000000000000 ) ) ;
#11209=DIRECTION ( 'NONE',  ( 1.000000000000000000, 0.000000000000000000, 0.000000000000000000 ) ) ;
#11230=ADVANCED_FACE ( 'NONE', ( #7130 ), #11632, .F. ) ;
#11237=ORIENTED_EDGE ( 'NONE', *, *, #2928, .T. ) ;
#11250=ORIENTED_EDGE ( 'NONE', *, *, #13223, .T. ) ;
#11251=VERTEX_POINT ( 'NONE', #2549 ) ;
#11257=DIRECTION ( 'NONE',  ( -1.000000000000000000, 0.000000000000000000, 0.000000000000000000 ) ) ;
#11268=AXIS2_PLACEMENT_3D ( 'NONE', #1730, #2920, #13495 ) ;
#11278=CIRCLE ( 'NONE', #5036, 1.000000000000000222 ) ;
#11279=CARTESIAN_POINT ( 'NONE',  ( -17.32050807568879236, -10.00000000000004263, 9.000000000000000000 ) ) ;
#11282=AXIS2_PLACEMENT_3D ( 'NONE', #4352, #14738, #17993 ) ;
#11285=EDGE_CURVE ( 'NONE', #9040, #7722, #5460, .T. ) ;
#11287=CARTESIAN_POINT ( 'NONE',  ( 2.449293598294706513E-15, -20.00000000000000000, 9.000000000000000000 ) ) ;
#11306=ORIENTED_EDGE ( 'NONE', *, *, #17333, .T. ) ;
#11315=LINE ( 'NONE', #7095, #14931 ) ;
#11327=EDGE_CURVE ( 'NONE', #3087, #8364, #18120, .T. ) ;
#11329=DIRECTION ( 'NONE',  ( 0.000000000000000000, -0.000000000000000000, 1.000000000000000000 ) ) ;
#11333=ORIENTED_EDGE ( 'NONE', *, *, #14293, .F. ) ;
#11338=DIRECTION ( 'NONE',  ( 0.000000000000000000, 0.000000000000000000, 1.000000000000000000 ) ) ;
#11347=EDGE_CURVE ( 'NONE', #258, #11140, #6306, .T. ) ;
#11348=DIRECTION ( 'NONE',  ( 1.000000000000000000, 0.000000000000000000, 0.000000000000000000 ) ) ;
#11350=DIRECTION ( 'NONE',  ( 0.000000000000000000, 0.000000000000000000, 1.000000000000000000 ) ) ;
#11353=ORIENTED_EDGE ( 'NONE', *, *, #7489, .T. ) ;
#11381=DIRECTION ( 'NONE',  ( 1.000000000000000000, 0.000000000000000000, 0.000000000000000000 ) ) ;
#11389=( NAMED_UNIT ( * ) SI_UNIT ( $, .STERADIAN. ) SOLID_ANGLE_UNIT ( ) );
#11394=CARTESIAN_POINT ( 'NONE',  ( -15.51323935927273645, -7.377028694403556131, 9.000000000000000000 ) ) ;
#11397=ORIENTED_EDGE ( 'NONE', *, *, #7357, .F. ) ;
#11405=VERTEX_POINT ( 'NONE', #10641 ) ;
#11410=AXIS2_PLACEMENT_3D ( 'NONE', #10383, #13231, #11748 ) ;
#11417=AXIS2_PLACEMENT_3D ( 'NONE', #19060, #18959, #1005 ) ;
#11420=ADVANCED_FACE ( 'NONE', ( #2923 ), #1542, .T. ) ;
#11430=ORIENTED_EDGE ( 'NONE', *, *, #6332, .T. ) ;
#11432=CARTESIAN_POINT ( 'NONE',  ( -14.86289650954781649, -33.38261212717723936, -9.000000000000000000 ) ) ;
#11440=DIRECTION ( 'NONE',  ( -0.000000000000000000, -0.000000000000000000, 1.000000000000000000 ) ) ;
#11443=LINE ( 'NONE', #14285, #8150 ) ;
#11453=ORIENTED_EDGE ( 'NONE', *, *, #16722, .F. ) ;
#11454=ORIENTED_EDGE ( 'NONE', *, *, #13837, .T. ) ;
#11455=DIRECTION ( 'NONE',  ( 0.000000000000000000, -0.000000000000000000, 1.000000000000000000 ) ) ;
#11461=CARTESIAN_POINT ( 'NONE',  ( 19.76107906696393357, -23.08216711247132835, 0.000000000000000000 ) ) ;
#11465=DIRECTION ( 'NONE',  ( -0.000000000000000000, -0.000000000000000000, -1.000000000000000000 ) ) ;
#11470=DIRECTION ( 'NONE',  ( 0.000000000000000000, 0.000000000000000000, 1.000000000000000000 ) ) ;
#11471=ADVANCED_FACE ( 'NONE', ( #17827 ), #4386, .F. ) ;
#11474=DIRECTION ( 'NONE',  ( -0.000000000000000000, -0.000000000000000000, -1.000000000000000000 ) ) ;
#11491=AXIS2_PLACEMENT_3D ( 'NONE', #12930, #13219, #5473 ) ;
#11493=LINE ( 'NONE', #15480, #5944 ) ;
#11520=ORIENTED_EDGE ( 'NONE', *, *, #14043, .T. ) ;
#11526=DIRECTION ( 'NONE',  ( -1.000000000000000000, 0.000000000000000000, 0.000000000000000000 ) ) ;
#11538=AXIS2_PLACEMENT_3D ( 'NONE', #7816, #383, #10946 ) ;
#11553=VERTEX_POINT ( 'NONE', #542 ) ;
#11554=EDGE_LOOP ( 'NONE', ( #5382, #3718, #3114, #13976 ) ) ;
#11555=DIRECTION ( 'NONE',  ( -0.6691306063588624564, 0.7431448254773903583, 0.000000000000000000 ) ) ;
#11577=FACE_OUTER_BOUND ( 'NONE', #15040, .T. ) ;
#11584=DIRECTION ( 'NONE',  ( 0.000000000000000000, -0.000000000000000000, 1.000000000000000000 ) ) ;
#11588=DIRECTION ( 'NONE',  ( 0.000000000000000000, 0.000000000000000000, 1.000000000000000000 ) ) ;
#11592=AXIS2_PLACEMENT_3D ( 'NONE', #15489, #17368, #1977 ) ;
#11594=CIRCLE ( 'NONE', #18823, 1.000000000000000000 ) ;
#11598=ORIENTED_EDGE ( 'NONE', *, *, #4544, .T. ) ;
#11599=CARTESIAN_POINT ( 'NONE',  ( 5.130877905917027526, -0.6693483836014323396, 9.000000000000000000 ) ) ;
#11602=CARTESIAN_POINT ( 'NONE',  ( -19.02113032590304442, -26.18033988749903074, -9.000000000000000000 ) ) ;
#11618=ORIENTED_EDGE ( 'NONE', *, *, #13341, .T. ) ;
#11619=ORIENTED_EDGE ( 'NONE', *, *, #17197, .F. ) ;
#11620=DIRECTION ( 'NONE',  ( -1.000000000000000000, 0.000000000000000000, 0.000000000000000000 ) ) ;
#11631=VERTEX_POINT ( 'NONE', #18695 ) ;
#11632=CYLINDRICAL_SURFACE ( 'NONE', #3183, 1.000000000000000000 ) ;
#11636=CYLINDRICAL_SURFACE ( 'NONE', #11168, 20.00000000000000000 ) ;
#11656=APPLICATION_CONTEXT ( 'automotive_design' ) ;
#11662=FACE_OUTER_BOUND ( 'NONE', #14142, .T. ) ;
#11665=EDGE_CURVE ( 'NONE', #12719, #15486, #5687, .T. ) ;
#11669=DIRECTION ( 'NONE',  ( 1.000000000000000000, 0.000000000000000000, 0.000000000000000000 ) ) ;
#11673=ORIENTED_EDGE ( 'NONE', *, *, #14578, .T. ) ;
#11679=LINE ( 'NONE', #10198, #17156 ) ;
#11690=CARTESIAN_POINT ( 'NONE',  ( 2.449293598294706513E-15, -20.00000000000000000, 9.000000000000000000 ) ) ;
#11695=VERTEX_POINT ( 'NONE', #6904 ) ;
#11714=FACE_OUTER_BOUND ( 'NONE', #10223, .T. ) ;
#11715=CARTESIAN_POINT ( 'NONE',  ( 2.449293598294706513E-15, -20.00000000000000000, 9.000000000000000000 ) ) ;
#11716=ORIENTED_EDGE ( 'NONE', *, *, #6162, .F. ) ;
#11717=ORIENTED_EDGE ( 'NONE', *, *, #17313, .F. ) ;
#11724=ORIENTED_EDGE ( 'NONE', *, *, #11119, .F. ) ;
#11731=CARTESIAN_POINT ( 'NONE',  ( -13.86289650954791064, -6.617387872822862782, -9.000000000000000000 ) ) ;
#11741=EDGE_LOOP ( 'NONE', ( #6535, #18066, #11673, #3900 ) ) ;
#11744=VERTEX_POINT ( 'NONE', #8271 ) ;
#11745=CARTESIAN_POINT ( 'NONE',  ( -19.89043790736545603, -22.09056926535314602, -9.000000000000000000 ) ) ;
#11748=DIRECTION ( 'NONE',  ( 0.3090169943749560000, -0.9510565162951507556, 0.000000000000000000 ) ) ;
#11756=CIRCLE ( 'NONE', #3325, 1.000000000000000444 ) ;
#11761=CARTESIAN_POINT ( 'NONE',  ( -8.134732861516020819, -1.729090847147989773, -9.000000000000000000 ) ) ;
#11790=VERTEX_POINT ( 'NONE', #18795 ) ;
#11792=EDGE_CURVE ( 'NONE', #14634, #12719, #11315, .T. ) ;
#11796=ORIENTED_EDGE ( 'NONE', *, *, #16480, .F. ) ;
#11800=PRODUCT ( 'driver roller', 'driver roller', '', ( #7749 ) ) ;
#11810=CARTESIAN_POINT ( 'NONE',  ( 2.449293598294706513E-15, -20.00000000000000000, 9.000000000000000000 ) ) ;
#11813=DIRECTION ( 'NONE',  ( 0.000000000000000000, 0.000000000000000000, -1.000000000000000000 ) ) ;
#11818=ORIENTED_EDGE ( 'NONE', *, *, #9328, .T. ) ;
#11826=CARTESIAN_POINT ( 'NONE',  ( -3.158233816355059620, -39.56295201467614220, 9.000000000000000000 ) ) ;
#11842=ORIENTED_EDGE ( 'NONE', *, *, #16042, .T. ) ;
#11847=FACE_OUTER_BOUND ( 'NONE', #637, .T. ) ;
#11859=DIRECTION ( 'NONE',  ( 0.000000000000000000, 0.000000000000000000, 1.000000000000000000 ) ) ;
#11863=DIRECTION ( 'NONE',  ( 0.000000000000000000, 0.000000000000000000, -1.000000000000000000 ) ) ;
#11870=DIRECTION ( 'NONE',  ( 1.000000000000000000, 0.000000000000000000, 0.000000000000000000 ) ) ;
#11871=CIRCLE ( 'NONE', #8436, 20.00000000000000000 ) ;
#11874=DIRECTION ( 'NONE',  ( -0.000000000000000000, -0.000000000000000000, -1.000000000000000000 ) ) ;
#11878=AXIS2_PLACEMENT_3D ( 'NONE', #6684, #14223, #17094 ) ;
#11887=CARTESIAN_POINT ( 'NONE',  ( -3.158233816355195955, -0.4370479853238878887, 9.000000000000000000 ) ) ;
#11903=AXIS2_PLACEMENT_3D ( 'NONE', #9873, #19026, #14579 ) ;
#11911=CARTESIAN_POINT ( 'NONE',  ( -18.68843350152494054, -12.87662627267948956, 9.000000000000000000 ) ) ;
#11930=FACE_OUTER_BOUND ( 'NONE', #18722, .T. ) ;
#11932=DIRECTION ( 'NONE',  ( 1.000000000000000000, 0.000000000000000000, 0.000000000000000000 ) ) ;
#11936=ORIENTED_EDGE ( 'NONE', *, *, #1841, .T. ) ;
#11945=DIRECTION ( 'NONE',  ( 0.000000000000000000, 0.000000000000000000, 1.000000000000000000 ) ) ;
#11952=CYLINDRICAL_SURFACE ( 'NONE', #8347, 1.000000000000000888 ) ;
#11953=EDGE_CURVE ( 'NONE', #6947, #2794, #8762, .T. ) ;
#11963=CARTESIAN_POINT ( 'NONE',  ( -18.68843350152494054, -12.87662627267948956, -9.000000000000000000 ) ) ;
#11968=ORIENTED_EDGE ( 'NONE', *, *, #13526, .F. ) ;
#11988=ADVANCED_BREP_SHAPE_REPRESENTATION ( '', ( #2528, #10359 ), #14982 ) ;
#11996=CARTESIAN_POINT ( 'NONE',  ( 2.449293598294706513E-15, -20.00000000000000000, -8.999999999999998224 ) ) ;
#11999=CARTESIAN_POINT ( 'NONE',  ( -19.97007065299860784, -21.09374499507130452, -9.000000000000000000 ) ) ;
#12007=VERTEX_POINT ( 'NONE', #17901 ) ;
#12015=ORIENTED_EDGE ( 'NONE', *, *, #9073, .T. ) ;
#12028=ADVANCED_FACE ( 'NONE', ( #12089 ), #1709, .T. ) ;
#12047=EDGE_CURVE ( 'NONE', #13178, #3535, #11152, .T. ) ;
#12054=DIRECTION ( 'NONE',  ( 0.000000000000000000, 0.000000000000000000, 1.000000000000000000 ) ) ;
#12059=DIRECTION ( 'NONE',  ( -0.000000000000000000, -0.000000000000000000, -1.000000000000000000 ) ) ;
#12063=VERTEX_POINT ( 'NONE', #6589 ) ;
#12065=CARTESIAN_POINT ( 'NONE',  ( 19.02113032590313679, -26.18033988749876428, 9.000000000000000000 ) ) ;
#12083=ORIENTED_EDGE ( 'NONE', *, *, #14903, .T. ) ;
#12087=DIRECTION ( 'NONE',  ( -1.000000000000000000, 0.000000000000000000, 0.000000000000000000 ) ) ;
#12089=FACE_OUTER_BOUND ( 'NONE', #5731, .T. ) ;
#12092=DIRECTION ( 'NONE',  ( 0.000000000000000000, 0.000000000000000000, 1.000000000000000000 ) ) ;
#12111=DIRECTION ( 'NONE',  ( 0.000000000000000000, 0.000000000000000000, 1.000000000000000000 ) ) ;
#12112=ORIENTED_EDGE ( 'NONE', *, *, #14214, .T. ) ;
#12121=ADVANCED_FACE ( 'NONE', ( #12572 ), #9432, .F. ) ;
#12130=AXIS2_PLACEMENT_3D ( 'NONE', #4332, #13250, #2881 ) ;
#12136=ADVANCED_FACE ( 'NONE', ( #17004 ), #1904, .F. ) ;
#12145=EDGE_CURVE ( 'NONE', #8857, #5700, #13055, .T. ) ;
#12162=AXIS2_PLACEMENT_3D ( 'NONE', #9491, #9302, #10682 ) ;
#12174=AXIS2_PLACEMENT_3D ( 'NONE', #14269, #18715, #15955 ) ;
#12176=VECTOR ( 'NONE', #2539, 1000.000000000000000 ) ;
#12178=ORIENTED_EDGE ( 'NONE', *, *, #5434, .F. ) ;
#12183=AXIS2_PLACEMENT_3D ( 'NONE', #16686, #7290, #13172 ) ;
#12185=DIRECTION ( 'NONE',  ( -0.000000000000000000, -0.000000000000000000, -1.000000000000000000 ) ) ;
#12201=DIRECTION ( 'NONE',  ( 1.000000000000000000, 0.000000000000000000, 0.000000000000000000 ) ) ;
#12217=DIRECTION ( 'NONE',  ( -0.9781476007338065770, 0.2079116908177552348, 0.000000000000000000 ) ) ;
#12220=AXIS2_PLACEMENT_3D ( 'NONE', #4383, #10637, #7512 ) ;
#12223=CIRCLE ( 'NONE', #10972, 20.00000000000000000 ) ;
#12230=CIRCLE ( 'NONE', #17258, 0.9999999999999991118 ) ;
#12233=AXIS2_PLACEMENT_3D ( 'NONE', #12992, #19001, #12903 ) ;
#12243=DIRECTION ( 'NONE',  ( 1.000000000000000000, 0.000000000000000000, 0.000000000000000000 ) ) ;
#12248=DIRECTION ( 'NONE',  ( 0.000000000000000000, -0.000000000000000000, -1.000000000000000000 ) ) ;
#12249=VECTOR ( 'NONE', #1153, 1000.000000000000000 ) ;
#12250=AXIS2_PLACEMENT_3D ( 'NONE', #18392, #348, #15050 ) ;
#12252=ORIENTED_EDGE ( 'NONE', *, *, #2609, .F. ) ;
#12266=CARTESIAN_POINT ( 'NONE',  ( 18.68843350152485527, -12.87662627267923909, 9.000000000000000000 ) ) ;
#12269=ADVANCED_FACE ( 'NONE', ( #5505 ), #7074, .F. ) ;
#12270=CARTESIAN_POINT ( 'NONE',  ( 1.000000000000000000, -14.00000000000000000, 8.999999999999998224 ) ) ;
#12277=DIRECTION ( 'NONE',  ( 1.000000000000000000, 0.000000000000000000, 0.000000000000000000 ) ) ;
#12287=CARTESIAN_POINT ( 'NONE',  ( -19.02113032590304442, -26.18033988749903074, 9.000000000000000000 ) ) ;
#12297=VERTEX_POINT ( 'NONE', #1201 ) ;
#12301=CARTESIAN_POINT ( 'NONE',  ( -8.134732861516020819, -1.729090847147989773, 9.000000000000000000 ) ) ;
#12303=ORIENTED_EDGE ( 'NONE', *, *, #1556, .T. ) ;
#12304=DIRECTION ( 'NONE',  ( 1.000000000000000000, 0.000000000000000000, 0.000000000000000000 ) ) ;
#12307=CARTESIAN_POINT ( 'NONE',  ( -19.89043790736545603, -22.09056926535314602, 9.000000000000000000 ) ) ;
#12315=DIRECTION ( 'NONE',  ( 0.000000000000000000, 0.000000000000000000, 1.000000000000000000 ) ) ;
#12318=EDGE_CURVE ( 'NONE', #6465, #6795, #17771, .T. ) ;
#12321=CARTESIAN_POINT ( 'NONE',  ( 14.86289650954800479, -33.38261212717704041, -9.000000000000000000 ) ) ;
#12323=EDGE_CURVE ( 'NONE', #18844, #12414, #4302, .T. ) ;
#12324=AXIS2_PLACEMENT_3D ( 'NONE', #14867, #10740, #1447 ) ;
#12327=VERTEX_POINT ( 'NONE', #8344 ) ;
#12328=AXIS2_PLACEMENT_3D ( 'NONE', #2199, #12473, #2099 ) ;
#12338=DIRECTION ( 'NONE',  ( -0.9135454576425982021, -0.4067366430758060925, 0.000000000000000000 ) ) ;
#12342=ORIENTED_EDGE ( 'NONE', *, *, #18456, .T. ) ;
#12355=VECTOR ( 'NONE', #4845, 1000.000000000000000 ) ;
#12366=EDGE_LOOP ( 'NONE', ( #5631, #10130, #4167, #2441 ) ) ;
#12371=ADVANCED_FACE ( 'NONE', ( #8641 ), #6875, .T. ) ;
#12386=CARTESIAN_POINT ( 'NONE',  ( -14.86289650954790886, -6.617387872822862782, 9.000000000000000000 ) ) ;
#12389=ORIENTED_EDGE ( 'NONE', *, *, #14534, .F. ) ;
#12390=FACE_OUTER_BOUND ( 'NONE', #10919, .T. ) ;
#12404=CARTESIAN_POINT ( 'NONE',  ( 2.449293598294706513E-15, -20.00000000000000000, 9.000000000000000000 ) ) ;
#12413=VERTEX_POINT ( 'NONE', #7274 ) ;
#12414=VERTEX_POINT ( 'NONE', #4234 ) ;
#12415=DIRECTION ( 'NONE',  ( -0.3090169943749528914, 0.9510565162951518658, 0.000000000000000000 ) ) ;
#12420=AXIS2_PLACEMENT_3D ( 'NONE', #13846, #10800, #8051 ) ;
#12433=DIRECTION ( 'NONE',  ( -0.8090169943749487835, 0.5877852522924713607, 0.000000000000000000 ) ) ;
#12456=DIRECTION ( 'NONE',  ( 0.000000000000000000, 0.000000000000000000, 1.000000000000000000 ) ) ;
#12468=VECTOR ( 'NONE', #10438, 1000.000000000000000 ) ;
#12473=DIRECTION ( 'NONE',  ( 0.000000000000000000, 0.000000000000000000, 1.000000000000000000 ) ) ;
#12488=ADVANCED_FACE ( 'NONE', ( #10299 ), #19265, .F. ) ;
#12496=EDGE_CURVE ( 'NONE', #8654, #12414, #11679, .T. ) ;
#12508=DIRECTION ( 'NONE',  ( 0.000000000000000000, 0.000000000000000000, -1.000000000000000000 ) ) ;
#12517=CYLINDRICAL_SURFACE ( 'NONE', #2798, 1.000000000000000888 ) ;
#12520=DIRECTION ( 'NONE',  ( 0.000000000000000000, 0.000000000000000000, 1.000000000000000000 ) ) ;
#12535=AXIS2_PLACEMENT_3D ( 'NONE', #2855, #10090, #14499 ) ;
#12539=ORIENTED_EDGE ( 'NONE', *, *, #8107, .F. ) ;
#12545=ORIENTED_EDGE ( 'NONE', *, *, #11327, .F. ) ;
#12552=DIRECTION ( 'NONE',  ( -0.000000000000000000, -0.000000000000000000, 1.000000000000000000 ) ) ;
#12572=FACE_OUTER_BOUND ( 'NONE', #13857, .T. ) ;
#12589=CIRCLE ( 'NONE', #3224, 20.00000000000000000 ) ;
#12600=CARTESIAN_POINT ( 'NONE',  ( -10.93224627749298605, -36.74771600333134103, 0.000000000000000000 ) ) ;
#12610=CARTESIAN_POINT ( 'NONE',  ( -10.75570504584937304, -36.18033988749900942, -9.000000000000000000 ) ) ;
#12618=EDGE_CURVE ( 'NONE', #15947, #4192, #3921, .T. ) ;
#12620=ORIENTED_EDGE ( 'NONE', *, *, #8813, .T. ) ;
#12626=EDGE_CURVE ( 'NONE', #5077, #15338, #3683, .T. ) ;
#12629=CARTESIAN_POINT ( 'NONE',  ( 17.32050807568866091, -9.999999999999797495, 9.000000000000000000 ) ) ;
#12634=ORIENTED_EDGE ( 'NONE', *, *, #9630, .T. ) ;
#12648=DIRECTION ( 'NONE',  ( 0.000000000000000000, 0.000000000000000000, 1.000000000000000000 ) ) ;
#12650=AXIS2_PLACEMENT_3D ( 'NONE', #4197, #13304, #10164 ) ;
#12657=CARTESIAN_POINT ( 'NONE',  ( 19.89043790736544892, -17.90943073464672608, -9.000000000000000000 ) ) ;
#12671=EDGE_CURVE ( 'NONE', #11107, #9525, #13994, .T. ) ;
#12683=VERTEX_POINT ( 'NONE', #5111 ) ;
#12693=EDGE_LOOP ( 'NONE', ( #17143, #16423, #15089, #14275 ) ) ;
#12710=CIRCLE ( 'NONE', #18991, 20.00000000000000000 ) ;
#12716=CIRCLE ( 'NONE', #3637, 1.000000000000001110 ) ;
#12719=VERTEX_POINT ( 'NONE', #18468 ) ;
#12725=DIRECTION ( 'NONE',  ( -0.000000000000000000, -0.000000000000000000, 1.000000000000000000 ) ) ;
#12727=DIRECTION ( 'NONE',  ( -0.000000000000000000, -0.000000000000000000, 1.000000000000000000 ) ) ;
#12733=VECTOR ( 'NONE', #2801, 1000.000000000000000 ) ;
#12737=DIRECTION ( 'NONE',  ( 0.000000000000000000, 0.000000000000000000, 1.000000000000000000 ) ) ;
#12756=DIRECTION ( 'NONE',  ( 0.000000000000000000, 0.000000000000000000, 1.000000000000000000 ) ) ;
#12777=CIRCLE ( 'NONE', #13410, 20.00000000000000000 ) ;
#12792=CIRCLE ( 'NONE', #4342, 0.9999999999999995559 ) ;
#12796=VERTEX_POINT ( 'NONE', #18954 ) ;
#12806=DIRECTION ( 'NONE',  ( -0.000000000000000000, -0.000000000000000000, 1.000000000000000000 ) ) ;
#12807=ORIENTED_EDGE ( 'NONE', *, *, #16972, .T. ) ;
#12810=ORIENTED_EDGE ( 'NONE', *, *, #176, .T. ) ;
#12816=ORIENTED_EDGE ( 'NONE', *, *, #2351, .F. ) ;
#12839=DIRECTION ( 'NONE',  ( 0.000000000000000000, 0.000000000000000000, 1.000000000000000000 ) ) ;
#12841=AXIS2_PLACEMENT_3D ( 'NONE', #1591, #117, #16691 ) ;
#12846=DIRECTION ( 'NONE',  ( 0.000000000000000000, 0.000000000000000000, 1.000000000000000000 ) ) ;
#12858=EDGE_CURVE ( 'NONE', #6513, #3553, #10000, .T. ) ;
#12866=CARTESIAN_POINT ( 'NONE',  ( -19.02113032590304442, -26.18033988749903074, -9.000000000000000000 ) ) ;
#12875=( NAMED_UNIT ( * ) PLANE_ANGLE_UNIT ( ) SI_UNIT ( $, .RADIAN. ) );
#12877=DIRECTION ( 'NONE',  ( 0.000000000000000000, 1.000000000000000000, 0.000000000000000000 ) ) ;
#12892=VERTEX_POINT ( 'NONE', #7165 ) ;
#12903=DIRECTION ( 'NONE',  ( -0.5000000000000041078, 0.8660254037844362651, 0.000000000000000000 ) ) ;
#12913=DIRECTION ( 'NONE',  ( 0.000000000000000000, 0.000000000000000000, 1.000000000000000000 ) ) ;
#12922=ADVANCED_FACE ( 'NONE', ( #5596 ), #17582, .F. ) ;
#12925=DIRECTION ( 'NONE',  ( 0.9781476007338055778, 0.2079116908177597867, 0.000000000000000000 ) ) ;
#12926=EDGE_CURVE ( 'NONE', #5570, #8337, #7768, .T. ) ;
#12930=CARTESIAN_POINT ( 'NONE',  ( -19.89043790736547379, -17.90943073464699609, -9.000000000000000000 ) ) ;
#12934=ORIENTED_EDGE ( 'NONE', *, *, #15447, .T. ) ;
#12935=EDGE_LOOP ( 'NONE', ( #15347, #4602, #11430, #2445 ) ) ;
#12945=CARTESIAN_POINT ( 'NONE',  ( -1.000000000000000000, -14.00000000000000000, 8.999999999999998224 ) ) ;
#12950=VECTOR ( 'NONE', #18606, 1000.000000000000000 ) ;
#12951=FACE_OUTER_BOUND ( 'NONE', #2221, .T. ) ;
#12954=CYLINDRICAL_SURFACE ( 'NONE', #17855, 20.00000000000000000 ) ;
#12956=ORIENTED_EDGE ( 'NONE', *, *, #6503, .F. ) ;
#12963=CARTESIAN_POINT ( 'NONE',  ( 2.449293598294706513E-15, -20.00000000000000000, 9.000000000000000000 ) ) ;
#12972=ORIENTED_EDGE ( 'NONE', *, *, #2201, .T. ) ;
#12974=EDGE_CURVE ( 'NONE', #15388, #1761, #9939, .T. ) ;
#12992=CARTESIAN_POINT ( 'NONE',  ( -17.32050807568872841, -30.00000000000008171, 9.000000000000000000 ) ) ;
#13005=CARTESIAN_POINT ( 'NONE',  ( -18.02113032590304442, -26.18033988749903074, -9.000000000000000000 ) ) ;
#13012=ORIENTED_EDGE ( 'NONE', *, *, #4788, .F. ) ;
#13023=DIRECTION ( 'NONE',  ( -1.000000000000000000, 0.000000000000000000, 0.000000000000000000 ) ) ;
#13026=AXIS2_PLACEMENT_3D ( 'NONE', #865, #14577, #11348 ) ;
#13027=LINE ( 'NONE', #19034, #2469 ) ;
#13028=ORIENTED_EDGE ( 'NONE', *, *, #10485, .F. ) ;
#13033=ADVANCED_FACE ( 'NONE', ( #1585 ), #10582, .T. ) ;
#13047=AXIS2_PLACEMENT_3D ( 'NONE', #12287, #4655, #233 ) ;
#13049=ORIENTED_EDGE ( 'NONE', *, *, #8553, .F. ) ;
#13053=DIRECTION ( 'NONE',  ( 0.000000000000000000, 0.000000000000000000, -1.000000000000000000 ) ) ;
#13055=CIRCLE ( 'NONE', #16189, 1.000000000000000000 ) ;
#13057=DIRECTION ( 'NONE',  ( 1.000000000000000000, 0.000000000000000000, 0.000000000000000000 ) ) ;
#13058=ORIENTED_EDGE ( 'NONE', *, *, #17206, .T. ) ;
#13069=ORIENTED_EDGE ( 'NONE', *, *, #8499, .T. ) ;
#13072=CARTESIAN_POINT ( 'NONE',  ( 2.449293598294706513E-15, -20.00000000000000000, 9.000000000000000000 ) ) ;
#13074=VERTEX_POINT ( 'NONE', #17969 ) ;
#13077=CARTESIAN_POINT ( 'NONE',  ( -14.86289650954790886, -6.617387872822862782, 9.000000000000000000 ) ) ;
#13078=ORIENTED_EDGE ( 'NONE', *, *, #15806, .F. ) ;
#13098=EDGE_CURVE ( 'NONE', #10464, #11251, #18118, .T. ) ;
#13115=CARTESIAN_POINT ( 'NONE',  ( 16.79901371501595975, -30.85325472854598416, -9.000000000000000000 ) ) ;
#13117=AXIS2_PLACEMENT_3D ( 'NONE', #12321, #15266, #274 ) ;
#13120=ORIENTED_EDGE ( 'NONE', *, *, #17798, .T. ) ;
#13121=ORIENTED_EDGE ( 'NONE', *, *, #3904, .F. ) ;
#13125=EDGE_CURVE ( 'NONE', #12007, #7897, #12777, .T. ) ;
#13126=CARTESIAN_POINT ( 'NONE',  ( 19.30627432446641123, -14.77814480204120784, 0.000000000000000000 ) ) ;
#13132=ORIENTED_EDGE ( 'NONE', *, *, #2839, .F. ) ;
#13133=DIRECTION ( 'NONE',  ( 1.000000000000000000, 0.000000000000000000, 0.000000000000000000 ) ) ;
#13151=AXIS2_PLACEMENT_3D ( 'NONE', #12065, #6285, #18068 ) ;
#13155=ORIENTED_EDGE ( 'NONE', *, *, #892, .F. ) ;
#13163=DIRECTION ( 'NONE',  ( 0.000000000000000000, 0.000000000000000000, 1.000000000000000000 ) ) ;
#13168=EDGE_CURVE ( 'NONE', #3999, #3553, #14808, .T. ) ;
#13172=DIRECTION ( 'NONE',  ( 1.000000000000000000, 0.000000000000000000, 0.000000000000000000 ) ) ;
#13178=VERTEX_POINT ( 'NONE', #6003 ) ;
#13182=AXIS2_PLACEMENT_3D ( 'NONE', #10855, #14278, #6446 ) ;
#13188=CIRCLE ( 'NONE', #4426, 20.00000000000000000 ) ;
#13194=ORIENTED_EDGE ( 'NONE', *, *, #14664, .F. ) ;
#13196=EDGE_LOOP ( 'NONE', ( #4593, #15657, #10317, #14085 ) ) ;
#13200=ORIENTED_EDGE ( 'NONE', *, *, #7704, .T. ) ;
#13203=VECTOR ( 'NONE', #7904, 1000.000000000000000 ) ;
#13216=ORIENTED_EDGE ( 'NONE', *, *, #6633, .T. ) ;
#13217=ORIENTED_EDGE ( 'NONE', *, *, #12671, .T. ) ;
#13219=DIRECTION ( 'NONE',  ( 0.000000000000000000, 0.000000000000000000, 1.000000000000000000 ) ) ;
#13223=EDGE_CURVE ( 'NONE', #1251, #4202, #7154, .T. ) ;
#13228=DIRECTION ( 'NONE',  ( 0.000000000000000000, 0.000000000000000000, 1.000000000000000000 ) ) ;
#13231=DIRECTION ( 'NONE',  ( 0.000000000000000000, 0.000000000000000000, 1.000000000000000000 ) ) ;
#13236=DIRECTION ( 'NONE',  ( -4.082155997157844188E-16, 1.000000000000000000, 0.000000000000000000 ) ) ;
#13248=LINE ( 'NONE', #16103, #5958 ) ;
#13250=DIRECTION ( 'NONE',  ( -0.000000000000000000, -0.000000000000000000, -1.000000000000000000 ) ) ;
#13269=DIRECTION ( 'NONE',  ( -0.5000000000000041078, 0.8660254037844362651, 0.000000000000000000 ) ) ;
#13273=ORIENTED_EDGE ( 'NONE', *, *, #13755, .F. ) ;
#13276=EDGE_CURVE ( 'NONE', #3696, #15553, #15602, .T. ) ;
#13279=DIRECTION ( 'NONE',  ( 0.000000000000000000, 0.000000000000000000, -1.000000000000000000 ) ) ;
#13294=FACE_OUTER_BOUND ( 'NONE', #6801, .T. ) ;
#13298=ORIENTED_EDGE ( 'NONE', *, *, #783, .F. ) ;
#13304=DIRECTION ( 'NONE',  ( 0.000000000000000000, 0.000000000000000000, 1.000000000000000000 ) ) ;
#13311=ORIENTED_EDGE ( 'NONE', *, *, #575, .T. ) ;
#13312=DIRECTION ( 'NONE',  ( -0.000000000000000000, 0.000000000000000000, 1.000000000000000000 ) ) ;
#13313=VECTOR ( 'NONE', #17873, 1000.000000000000000 ) ;
#13317=DIRECTION ( 'NONE',  ( -0.000000000000000000, -0.000000000000000000, -1.000000000000000000 ) ) ;
#13319=EDGE_LOOP ( 'NONE', ( #15515, #256, #3106, #18121, #14860, #6368 ) ) ;
#13320=CYLINDRICAL_SURFACE ( 'NONE', #13794, 1.000000000000000888 ) ;
#13338=EDGE_CURVE ( 'NONE', #18235, #14101, #2160, .T. ) ;
#13339=ADVANCED_FACE ( 'NONE', ( #686 ), #6657, .T. ) ;
#13340=DIRECTION ( 'NONE',  ( 0.000000000000000000, 0.000000000000000000, 1.000000000000000000 ) ) ;
#13341=EDGE_CURVE ( 'NONE', #14650, #12327, #15921, .T. ) ;
#13347=ADVANCED_FACE ( 'NONE', ( #4812 ), #10776, .T. ) ;
#13366=ORIENTED_EDGE ( 'NONE', *, *, #17739, .F. ) ;
#13370=ORIENTED_EDGE ( 'NONE', *, *, #9863, .F. ) ;
#13372=DIRECTION ( 'NONE',  ( 1.000000000000000000, 0.000000000000000000, -0.000000000000000000 ) ) ;
#13374=DIRECTION ( 'NONE',  ( -0.000000000000000000, -0.000000000000000000, 1.000000000000000000 ) ) ;
#13388=CARTESIAN_POINT ( 'NONE',  ( -19.89043790736547379, -17.90943073464699609, -9.000000000000000000 ) ) ;
#13392=DIRECTION ( 'NONE',  ( 0.000000000000000000, 0.000000000000000000, 1.000000000000000000 ) ) ;
#13396=ORIENTED_EDGE ( 'NONE', *, *, #5083, .F. ) ;
#13400=CARTESIAN_POINT ( 'NONE',  ( -10.75570504584948139, -3.819660112501066518, 9.000000000000000000 ) ) ;
#13410=AXIS2_PLACEMENT_3D ( 'NONE', #10190, #16190, #14705 ) ;
#13424=CIRCLE ( 'NONE', #18771, 0.9999999999999993339 ) ;
#13427=FACE_OUTER_BOUND ( 'NONE', #2599, .T. ) ;
#13438=CARTESIAN_POINT ( 'NONE',  ( -0.9999999999999976685, -20.00000000000000000, -9.000000000000001776 ) ) ;
#13441=CIRCLE ( 'NONE', #9998, 20.00000000000000000 ) ;
#13444=DIRECTION ( 'NONE',  ( -0.000000000000000000, -0.000000000000000000, -1.000000000000000000 ) ) ;
#13459=ADVANCED_FACE ( 'NONE', ( #871 ), #2563, .T. ) ;
#13464=ADVANCED_FACE ( 'NONE', ( #17552 ), #10079, .F. ) ;
#13469=EDGE_CURVE ( 'NONE', #3609, #5700, #19075, .T. ) ;
#13471=CIRCLE ( 'NONE', #4709, 1.000000000000000888 ) ;
#13473=ORIENTED_EDGE ( 'NONE', *, *, #12858, .T. ) ;
#13479=AXIS2_PLACEMENT_3D ( 'NONE', #6138, #3117, #1249 ) ;
#13484=CIRCLE ( 'NONE', #8774, 1.000000000000001110 ) ;
#13494=ORIENTED_EDGE ( 'NONE', *, *, #6221, .F. ) ;
#13495=DIRECTION ( 'NONE',  ( -1.000000000000000000, 0.000000000000000000, 0.000000000000000000 ) ) ;
#13499=CARTESIAN_POINT ( 'NONE',  ( -7.134732861516020819, -1.729090847147989773, -9.000000000000000000 ) ) ;
#13503=AXIS2_PLACEMENT_3D ( 'NONE', #17401, #12877, #2305 ) ;
#13516=DIRECTION ( 'NONE',  ( 0.000000000000000000, 0.000000000000000000, 1.000000000000000000 ) ) ;
#13526=EDGE_CURVE ( 'NONE', #7511, #2842, #5972, .T. ) ;
#13538=CARTESIAN_POINT ( 'NONE',  ( 2.449293598294706513E-15, -20.00000000000000000, 9.000000000000000000 ) ) ;
#13540=CARTESIAN_POINT ( 'NONE',  ( 2.449293598294706513E-15, -20.00000000000000000, 9.000000000000000000 ) ) ;
#13551=DIRECTION ( 'NONE',  ( 0.000000000000000000, 0.000000000000000000, 1.000000000000000000 ) ) ;
#13561=ORIENTED_EDGE ( 'NONE', *, *, #12496, .T. ) ;
#13570=DIRECTION ( 'NONE',  ( 0.000000000000000000, 0.000000000000000000, 1.000000000000000000 ) ) ;
#13577=ORIENTED_EDGE ( 'NONE', *, *, #2409, .T. ) ;
#13591=AXIS2_PLACEMENT_3D ( 'NONE', #1790, #13551, #16407 ) ;
#13597=DIRECTION ( 'NONE',  ( 1.000000000000000000, 0.000000000000000000, 0.000000000000000000 ) ) ;
#13605=VECTOR ( 'NONE', #2578, 1000.000000000000000 ) ;
#13608=ORIENTED_EDGE ( 'NONE', *, *, #9442, .T. ) ;
#13640=CARTESIAN_POINT ( 'NONE',  ( 2.449293598294706513E-15, -20.00000000000000000, 9.000000000000000000 ) ) ;
#13657=CARTESIAN_POINT ( 'NONE',  ( 2.449293598294706513E-15, -20.00000000000000000, 9.000000000000000000 ) ) ;
#13660=DIRECTION ( 'NONE',  ( 1.000000000000000000, 0.000000000000000000, 0.000000000000000000 ) ) ;
#13673=LINE ( 'NONE', #5046, #1236 ) ;
#13683=AXIS2_PLACEMENT_3D ( 'NONE', #6782, #9909, #11381 ) ;
#13692=EDGE_CURVE ( 'NONE', #3574, #11631, #2039, .T. ) ;
#13701=CARTESIAN_POINT ( 'NONE',  ( 15.51323935927256237, -7.377028694403341191, -9.000000000000000000 ) ) ;
#13702=EDGE_LOOP ( 'NONE', ( #12252, #3016, #17023, #14636 ) ) ;
#13719=EDGE_CURVE ( 'NONE', #18444, #6580, #13424, .T. ) ;
#13721=CARTESIAN_POINT ( 'NONE',  ( 1.000000000000002442, -20.00000000000000000, 8.999999999999998224 ) ) ;
#13728=CARTESIAN_POINT ( 'NONE',  ( -4.999999999999998224, -20.00000000000000000, 15.00000000000000355 ) ) ;
#13745=ORIENTED_EDGE ( 'NONE', *, *, #1871, .F. ) ;
#13755=EDGE_CURVE ( 'NONE', #6465, #16560, #10605, .T. ) ;
#13765=ORIENTED_EDGE ( 'NONE', *, *, #13168, .F. ) ;
#13771=ORIENTED_EDGE ( 'NONE', *, *, #6329, .T. ) ;
#13772=DIRECTION ( 'NONE',  ( -1.000000000000000000, 0.000000000000000000, 0.000000000000000000 ) ) ;
#13783=VECTOR ( 'NONE', #14188, 1000.000000000000000 ) ;
#13784=AXIS2_PLACEMENT_3D ( 'NONE', #2219, #6417, #13772 ) ;
#13789=FACE_OUTER_BOUND ( 'NONE', #8451, .T. ) ;
#13794=AXIS2_PLACEMENT_3D ( 'NONE', #11745, #11455, #13133 ) ;
#13800=CYLINDRICAL_SURFACE ( 'NONE', #2067, 20.00000000000000000 ) ;
#13810=CARTESIAN_POINT ( 'NONE',  ( -19.89043790736545603, -22.09056926535314602, 9.000000000000000000 ) ) ;
#13813=VECTOR ( 'NONE', #1829, 1000.000000000000000 ) ;
#13814=CIRCLE ( 'NONE', #5365, 0.9999999999999991118 ) ;
#13819=VERTEX_POINT ( 'NONE', #7999 ) ;
#13824=CARTESIAN_POINT ( 'NONE',  ( 0.9996874511566150590, -39.97499999999999432, 0.000000000000000000 ) ) ;
#13837=EDGE_CURVE ( 'NONE', #11082, #1055, #14349, .T. ) ;
#13846=CARTESIAN_POINT ( 'NONE',  ( -17.32050807568879236, -10.00000000000004263, -9.000000000000000000 ) ) ;
#13848=DIRECTION ( 'NONE',  ( -0.000000000000000000, -0.000000000000000000, -1.000000000000000000 ) ) ;
#13857=EDGE_LOOP ( 'NONE', ( #1608, #1968, #673, #17640 ) ) ;
#13867=VERTEX_POINT ( 'NONE', #12610 ) ;
#13874=CARTESIAN_POINT ( 'NONE',  ( -7.134732861516020819, -1.729090847147989773, 9.000000000000000000 ) ) ;
#13878=CARTESIAN_POINT ( 'NONE',  ( 2.449293598294706513E-15, -20.00000000000000000, -9.000000000000000000 ) ) ;
#13885=AXIS2_PLACEMENT_3D ( 'NONE', #18486, #17103, #3757 ) ;
#13898=VECTOR ( 'NONE', #11073, 1000.000000000000000 ) ;
#13901=ORIENTED_EDGE ( 'NONE', *, *, #14789, .F. ) ;
#13913=CARTESIAN_POINT ( 'NONE',  ( 14.86289650954772590, -6.617387872822656725, -9.000000000000000000 ) ) ;
#13925=AXIS2_PLACEMENT_3D ( 'NONE', #11066, #5184, #11257 ) ;
#13932=CARTESIAN_POINT ( 'NONE',  ( -4.158233816355195955, -0.4370479853238878887, -9.000000000000000000 ) ) ;
#13945=EDGE_CURVE ( 'NONE', #11405, #3727, #1051, .T. ) ;
#13951=ORIENTED_EDGE ( 'NONE', *, *, #6503, .T. ) ;
#13957=DIRECTION ( 'NONE',  ( 1.000000000000000000, 0.000000000000000000, 0.000000000000000000 ) ) ;
#13967=CARTESIAN_POINT ( 'NONE',  ( 9.037824375505316254, -2.158539001597377105, 9.000000000000000000 ) ) ;
#13976=ORIENTED_EDGE ( 'NONE', *, *, #17812, .T. ) ;
#13979=EDGE_LOOP ( 'NONE', ( #15177, #10668, #630, #9956 ) ) ;
#13981=ORIENTED_EDGE ( 'NONE', *, *, #16972, .F. ) ;
#13990=CARTESIAN_POINT ( 'NONE',  ( -16.32050807568872841, -30.00000000000008171, -9.000000000000000000 ) ) ;
#13994=CIRCLE ( 'NONE', #5553, 0.9999999999999985567 ) ;
#14003=DIRECTION ( 'NONE',  ( 1.000000000000000000, 0.000000000000000000, 0.000000000000000000 ) ) ;
#14007=DIRECTION ( 'NONE',  ( 0.000000000000000000, 0.000000000000000000, 1.000000000000000000 ) ) ;
#14022=EDGE_LOOP ( 'NONE', ( #5726, #13273, #15852, #17451 ) ) ;
#14027=VERTEX_POINT ( 'NONE', #661 ) ;
#14043=EDGE_CURVE ( 'NONE', #11186, #17731, #12792, .T. ) ;
#14051=ORIENTED_EDGE ( 'NONE', *, *, #6565, .T. ) ;
#14059=CARTESIAN_POINT ( 'NONE',  ( -7.134732861515892033, -38.27090915285207018, -9.000000000000000000 ) ) ;
#14063=ADVANCED_FACE ( 'NONE', ( #1144 ), #1435, .T. ) ;
#14084=AXIS2_PLACEMENT_3D ( 'NONE', #6706, #5048, #12304 ) ;
#14085=ORIENTED_EDGE ( 'NONE', *, *, #14954, .F. ) ;
#14089=CARTESIAN_POINT ( 'NONE',  ( 17.32050807568887052, -29.99999999999984013, -9.000000000000000000 ) ) ;
#14093=VECTOR ( 'NONE', #6652, 1000.000000000000000 ) ;
#14098=DIRECTION ( 'NONE',  ( 0.000000000000000000, 0.000000000000000000, 1.000000000000000000 ) ) ;
#14101=VERTEX_POINT ( 'NONE', #11911 ) ;
#14103=EDGE_CURVE ( 'NONE', #6513, #2794, #5946, .T. ) ;
#14105=ORIENTED_EDGE ( 'NONE', *, *, #18888, .F. ) ;
#14107=EDGE_CURVE ( 'NONE', #5700, #8510, #3008, .T. ) ;
#14121=EDGE_LOOP ( 'NONE', ( #10313, #5517, #6248, #13049 ) ) ;
#14142=EDGE_LOOP ( 'NONE', ( #975, #2632, #7775, #2912 ) ) ;
#14148=CIRCLE ( 'NONE', #1971, 1.000000000000000222 ) ;
#14154=ORIENTED_EDGE ( 'NONE', *, *, #1987, .F. ) ;
#14168=ORIENTED_EDGE ( 'NONE', *, *, #16859, .T. ) ;
#14181=ORIENTED_EDGE ( 'NONE', *, *, #12926, .T. ) ;
#14188=DIRECTION ( 'NONE',  ( 0.000000000000000000, -0.000000000000000000, 1.000000000000000000 ) ) ;
#14189=AXIS2_PLACEMENT_3D ( 'NONE', #12404, #11026, #16933 ) ;
#14191=ORIENTED_EDGE ( 'NONE', *, *, #1733, .T. ) ;
#14197=ORIENTED_EDGE ( 'NONE', *, *, #5822, .T. ) ;
#14198=DIRECTION ( 'NONE',  ( -0.5000000000000041078, 0.8660254037844362651, 0.000000000000000000 ) ) ;
#14200=ORIENTED_EDGE ( 'NONE', *, *, #6749, .T. ) ;
#14201=AXIS2_PLACEMENT_3D ( 'NONE', #2120, #6517, #9358 ) ;
#14202=DIRECTION ( 'NONE',  ( 0.000000000000000000, 0.000000000000000000, 1.000000000000000000 ) ) ;
#14205=CIRCLE ( 'NONE', #12328, 20.00000000000000000 ) ;
#14207=CARTESIAN_POINT ( 'NONE',  ( -14.17539641854911281, -34.10879641843998655, 0.000000000000000000 ) ) ;
#14209=DIRECTION ( 'NONE',  ( -0.000000000000000000, -0.000000000000000000, 1.000000000000000000 ) ) ;
#14212=CARTESIAN_POINT ( 'NONE',  ( 2.449293598294706513E-15, -20.00000000000000000, 9.000000000000000000 ) ) ;
#14214=EDGE_CURVE ( 'NONE', #258, #7750, #2728, .T. ) ;
#14217=AXIS2_PLACEMENT_3D ( 'NONE', #19267, #214, #5806 ) ;
#14218=CARTESIAN_POINT ( 'NONE',  ( 17.79870116617255604, -29.12174527145369396, 9.000000000000000000 ) ) ;
#14223=DIRECTION ( 'NONE',  ( 0.000000000000000000, 0.000000000000000000, 1.000000000000000000 ) ) ;
#14231=CYLINDRICAL_SURFACE ( 'NONE', #8247, 1.000000000000000888 ) ;
#14243=CARTESIAN_POINT ( 'NONE',  ( -19.97007065299860784, -21.09374499507130452, 0.000000000000000000 ) ) ;
#14246=ORIENTED_EDGE ( 'NONE', *, *, #10149, .T. ) ;
#14247=DIRECTION ( 'NONE',  ( -0.3090169943749528914, 0.9510565162951518658, 0.000000000000000000 ) ) ;
#14249=ORIENTED_EDGE ( 'NONE', *, *, #1860, .T. ) ;
#14263=CARTESIAN_POINT ( 'NONE',  ( -18.68843350152488725, -27.12337372732065077, -9.000000000000000000 ) ) ;
#14265=ORIENTED_EDGE ( 'NONE', *, *, #11792, .F. ) ;
#14269=CARTESIAN_POINT ( 'NONE',  ( 2.449293598294706513E-15, -20.00000000000000000, 9.000000000000000000 ) ) ;
#14275=ORIENTED_EDGE ( 'NONE', *, *, #7935, .F. ) ;
#14277=ORIENTED_EDGE ( 'NONE', *, *, #9368, .F. ) ;
#14278=DIRECTION ( 'NONE',  ( 0.000000000000000000, 0.000000000000000000, 1.000000000000000000 ) ) ;
#14285=CARTESIAN_POINT ( 'NONE',  ( -18.02113032590308705, -13.81966011250110249, -9.000000000000000000 ) ) ;
#14293=EDGE_CURVE ( 'NONE', #8366, #8685, #3424, .T. ) ;
#14307=ADVANCED_FACE ( 'NONE', ( #12390 ), #4670, .F. ) ;
#14308=CYLINDRICAL_SURFACE ( 'NONE', #1182, 0.9999999999999991118 ) ;
#14319=DIRECTION ( 'NONE',  ( -0.000000000000000000, -0.000000000000000000, -1.000000000000000000 ) ) ;
#14328=CARTESIAN_POINT ( 'NONE',  ( -4.158233816355060064, -39.56295201467614220, -9.000000000000000000 ) ) ;
#14339=COLOUR_RGB ( '',0.8941176470588234615, 0.8941176470588234615, 0.8941176470588234615 ) ;
#14345=CYLINDRICAL_SURFACE ( 'NONE', #4424, 0.9999999999999991118 ) ;
#14349=CIRCLE ( 'NONE', #13117, 1.000000000000002665 ) ;
#14350=ORIENTED_EDGE ( 'NONE', *, *, #1841, .F. ) ;
#14358=LINE ( 'NONE', #12600, #1816 ) ;
#14364=ORIENTED_EDGE ( 'NONE', *, *, #15493, .T. ) ;
#14366=ORIENTED_EDGE ( 'NONE', *, *, #18497, .F. ) ;
#14378=AXIS2_PLACEMENT_3D ( 'NONE', #16031, #14451, #11207 ) ;
#14382=LINE ( 'NONE', #5082, #4290 ) ;
#14387=LINE ( 'NONE', #6741, #15666 ) ;
#14397=AXIS2_PLACEMENT_3D ( 'NONE', #8382, #2631, #5356 ) ;
#14408=AXIS2_PLACEMENT_3D ( 'NONE', #4199, #8703, #6065 ) ;
#14430=DIRECTION ( 'NONE',  ( 0.000000000000000000, -0.000000000000000000, 1.000000000000000000 ) ) ;
#14434=EDGE_CURVE ( 'NONE', #8760, #15486, #2110, .T. ) ;
#14435=FACE_OUTER_BOUND ( 'NONE', #17020, .T. ) ;
#14442=EDGE_CURVE ( 'NONE', #16376, #7688, #5926, .T. ) ;
#14451=DIRECTION ( 'NONE',  ( -9.858538378746663627E-23, 5.031452844637890958E-23, -1.000000000000000000 ) ) ;
#14452=ORIENTED_EDGE ( 'NONE', *, *, #8720, .F. ) ;
#14459=CARTESIAN_POINT ( 'NONE',  ( 1.000000000000002442, -20.00000000000000000, -9.000000000000001776 ) ) ;
#14463=AXIS2_PLACEMENT_3D ( 'NONE', #791, #17732, #695 ) ;
#14464=CARTESIAN_POINT ( 'NONE',  ( -19.99999999999999645, -20.00000000000000000, -9.000000000000000000 ) ) ;
#14479=DIRECTION ( 'NONE',  ( 0.9135454576426006446, 0.4067366430758008189, 0.000000000000000000 ) ) ;
#14482=ORIENTED_EDGE ( 'NONE', *, *, #9868, .F. ) ;
#14486=DIRECTION ( 'NONE',  ( 0.000000000000000000, 0.000000000000000000, 1.000000000000000000 ) ) ;
#14491=ORIENTED_EDGE ( 'NONE', *, *, #6215, .F. ) ;
#14497=ORIENTED_EDGE ( 'NONE', *, *, #10705, .T. ) ;
#14499=DIRECTION ( 'NONE',  ( -1.000000000000000000, 0.000000000000000000, 0.000000000000000000 ) ) ;
#14503=DIRECTION ( 'NONE',  ( 0.000000000000000000, 0.000000000000000000, 1.000000000000000000 ) ) ;
#14505=LINE ( 'NONE', #11461, #6319 ) ;
#14515=CARTESIAN_POINT ( 'NONE',  ( -13.86289650954791064, -6.617387872822862782, 9.000000000000000000 ) ) ;
#14517=DIRECTION ( 'NONE',  ( -0.000000000000000000, -0.000000000000000000, -1.000000000000000000 ) ) ;
#14527=CYLINDRICAL_SURFACE ( 'NONE', #15038, 1.000000000000000000 ) ;
#14530=ADVANCED_FACE ( 'NONE', ( #18686 ), #18885, .F. ) ;
#14532=CARTESIAN_POINT ( 'NONE',  ( 2.449293598294706513E-15, -20.00000000000000000, 9.000000000000000000 ) ) ;
#14533=ORIENTED_EDGE ( 'NONE', *, *, #2351, .T. ) ;
#14534=EDGE_CURVE ( 'NONE', #6336, #12413, #10303, .T. ) ;
#14535=EDGE_CURVE ( 'NONE', #5652, #3609, #8264, .T. ) ;
#14550=VECTOR ( 'NONE', #14319, 1000.000000000000000 ) ;
#14556=ORIENTED_EDGE ( 'NONE', *, *, #8089, .T. ) ;
#14558=ORIENTED_EDGE ( 'NONE', *, *, #18402, .F. ) ;
#14568=VERTEX_POINT ( 'NONE', #19280 ) ;
#14577=DIRECTION ( 'NONE',  ( 0.000000000000000000, 0.000000000000000000, 1.000000000000000000 ) ) ;
#14578=EDGE_CURVE ( 'NONE', #11631, #7961, #911, .T. ) ;
#14579=DIRECTION ( 'NONE',  ( 1.000000000000000000, 0.000000000000000000, 0.000000000000000000 ) ) ;
#14584=CARTESIAN_POINT ( 'NONE',  ( 2.449293598294706513E-15, -20.00000000000000000, 9.000000000000000000 ) ) ;
#14587=DIRECTION ( 'NONE',  ( 0.000000000000000000, -0.000000000000000000, 1.000000000000000000 ) ) ;
#14589=CARTESIAN_POINT ( 'NONE',  ( -19.02113032590308705, -13.81966011250110249, 9.000000000000000000 ) ) ;
#14597=ADVANCED_FACE ( 'NONE', ( #5818 ), #2793, .T. ) ;
#14604=CARTESIAN_POINT ( 'NONE',  ( 2.449293598294706513E-15, -20.00000000000000000, -9.000000000000000000 ) ) ;
#14632=DIRECTION ( 'NONE',  ( 0.000000000000000000, 0.000000000000000000, 1.000000000000000000 ) ) ;
#14633=EDGE_CURVE ( 'NONE', #19111, #10629, #16895, .T. ) ;
#14634=VERTEX_POINT ( 'NONE', #3252 ) ;
#14636=ORIENTED_EDGE ( 'NONE', *, *, #8089, .F. ) ;
#14643=DIRECTION ( 'NONE',  ( 1.000000000000000000, 0.000000000000000000, 0.000000000000000000 ) ) ;
#14644=CARTESIAN_POINT ( 'NONE',  ( -17.79870116617242459, -29.12174527145394265, 0.000000000000000000 ) ) ;
#14648=FACE_OUTER_BOUND ( 'NONE', #3679, .T. ) ;
#14650=VERTEX_POINT ( 'NONE', #10213 ) ;
#14654=CARTESIAN_POINT ( 'NONE',  ( 2.449293598294706513E-15, -20.00000000000000000, 9.000000000000000000 ) ) ;
#14661=ORIENTED_EDGE ( 'NONE', *, *, #10804, .T. ) ;
#14664=EDGE_CURVE ( 'NONE', #16610, #18021, #13441, .T. ) ;
#14666=EDGE_CURVE ( 'NONE', #18444, #1643, #11871, .T. ) ;
#14667=ORIENTED_EDGE ( 'NONE', *, *, #13098, .F. ) ;
#14682=EDGE_CURVE ( 'NONE', #9693, #8618, #11493, .T. ) ;
#14683=ORIENTED_EDGE ( 'NONE', *, *, #13168, .T. ) ;
#14705=DIRECTION ( 'NONE',  ( 1.000000000000000000, 0.000000000000000000, 0.000000000000000000 ) ) ;
#14709=VECTOR ( 'NONE', #12806, 1000.000000000000000 ) ;
#14719=CIRCLE ( 'NONE', #6894, 1.000000000000000000 ) ;
#14726=CARTESIAN_POINT ( 'NONE',  ( 19.02113032590313679, -26.18033988749876428, -9.000000000000000000 ) ) ;
#14730=EDGE_LOOP ( 'NONE', ( #4481, #924, #14732, #16833 ) ) ;
#14732=ORIENTED_EDGE ( 'NONE', *, *, #10215, .T. ) ;
#14733=CARTESIAN_POINT ( 'NONE',  ( 2.449293598294706513E-15, -20.00000000000000000, -9.000000000000000000 ) ) ;
#14738=DIRECTION ( 'NONE',  ( -0.000000000000000000, -0.000000000000000000, 1.000000000000000000 ) ) ;
#14755=ORIENTED_EDGE ( 'NONE', *, *, #16480, .T. ) ;
#14768=CARTESIAN_POINT ( 'NONE',  ( 10.93224627749321876, -36.74771600333119181, 9.000000000000000000 ) ) ;
#14777=EDGE_CURVE ( 'NONE', #12892, #2842, #3442, .T. ) ;
#14789=EDGE_CURVE ( 'NONE', #17065, #4767, #7504, .T. ) ;
#14797=CARTESIAN_POINT ( 'NONE',  ( 2.449293598294706513E-15, -20.00000000000000000, 9.000000000000000000 ) ) ;
#14808=LINE ( 'NONE', #13438, #6825 ) ;
#14812=ORIENTED_EDGE ( 'NONE', *, *, #19295, .T. ) ;
#14813=PLANE ( 'NONE',  #11417 ) ;
#14822=CYLINDRICAL_SURFACE ( 'NONE', #5688, 5.000000000000000888 ) ;
#14831=EDGE_CURVE ( 'NONE', #7722, #8295, #3713, .T. ) ;
#14860=ORIENTED_EDGE ( 'NONE', *, *, #14103, .T. ) ;
#14867=CARTESIAN_POINT ( 'NONE',  ( -8.134732861515892921, -38.27090915285207018, -9.000000000000000000 ) ) ;
#14872=CARTESIAN_POINT ( 'NONE',  ( 11.75570504584960041, -36.18033988749885310, 9.000000000000000000 ) ) ;
#14873=CARTESIAN_POINT ( 'NONE',  ( 19.02113032590300890, -13.81966011250085025, 9.000000000000000000 ) ) ;
#14881=AXIS2_PLACEMENT_3D ( 'NONE', #1973, #15483, #14198 ) ;
#14897=EDGE_CURVE ( 'NONE', #16610, #11107, #13027, .T. ) ;
#14898=DIRECTION ( 'NONE',  ( 1.000000000000000000, -6.938893903907227392E-16, 0.000000000000000000 ) ) ;
#14903=EDGE_CURVE ( 'NONE', #666, #3752, #2463, .T. ) ;
#14911=ORIENTED_EDGE ( 'NONE', *, *, #934, .F. ) ;
#14918=DIRECTION ( 'NONE',  ( 0.6691306063588675634, -0.7431448254773859174, 0.000000000000000000 ) ) ;
#14919=FACE_OUTER_BOUND ( 'NONE', #16739, .T. ) ;
#14920=CYLINDRICAL_SURFACE ( 'NONE', #3680, 1.000000000000000888 ) ;
#14922=LINE ( 'NONE', #7761, #4821 ) ;
#14929=ORIENTED_EDGE ( 'NONE', *, *, #15493, .F. ) ;
#14931=VECTOR ( 'NONE', #2619, 1000.000000000000000 ) ;
#14934=ORIENTED_EDGE ( 'NONE', *, *, #2382, .F. ) ;
#14943=CARTESIAN_POINT ( 'NONE',  ( -18.68843350152489080, -27.12337372732064011, 0.000000000000000000 ) ) ;
#14954=EDGE_CURVE ( 'NONE', #15438, #18021, #3827, .T. ) ;
#14957=VECTOR ( 'NONE', #6670, 1000.000000000000000 ) ;
#14970=DIRECTION ( 'NONE',  ( 0.000000000000000000, 0.000000000000000000, 1.000000000000000000 ) ) ;
#14982=( GEOMETRIC_REPRESENTATION_CONTEXT ( 3 ) GLOBAL_UNCERTAINTY_ASSIGNED_CONTEXT ( ( #9482 ) ) GLOBAL_UNIT_ASSIGNED_CONTEXT ( ( #399, #17265, #583 ) ) REPRESENTATION_CONTEXT ( 'NONE', 'WORKASPACE' ) );
#14983=VERTEX_POINT ( 'NONE', #1365 ) ;
#14994=CARTESIAN_POINT ( 'NONE',  ( 19.89043790736549155, -22.09056926535286891, -9.000000000000000000 ) ) ;
#15001=DIRECTION ( 'NONE',  ( -1.000000000000000000, 0.000000000000000000, 0.000000000000000000 ) ) ;
#15002=EDGE_LOOP ( 'NONE', ( #8371, #10952, #18711, #14934 ) ) ;
#15006=EDGE_CURVE ( 'NONE', #11790, #1052, #2787, .T. ) ;
#15007=AXIS2_PLACEMENT_3D ( 'NONE', #13072, #2613, #10028 ) ;
#15013=CARTESIAN_POINT ( 'NONE',  ( 9.037824375505676855, -37.84146099840244659, 9.000000000000000000 ) ) ;
#15025=VECTOR ( 'NONE', #7554, 1000.000000000000000 ) ;
#15038=AXIS2_PLACEMENT_3D ( 'NONE', #8462, #1113, #15923 ) ;
#15040=EDGE_LOOP ( 'NONE', ( #12389, #1166, #15156, #15957 ) ) ;
#15041=CARTESIAN_POINT ( 'NONE',  ( -4.158233816355060064, -39.56295201467614220, -9.000000000000000000 ) ) ;
#15050=DIRECTION ( 'NONE',  ( -1.000000000000000000, 0.000000000000000000, 0.000000000000000000 ) ) ;
#15054=ORIENTED_EDGE ( 'NONE', *, *, #3404, .F. ) ;
#15061=CARTESIAN_POINT ( 'NONE',  ( -13.86289650954791064, -6.617387872822862782, -9.000000000000000000 ) ) ;
#15080=ORIENTED_EDGE ( 'NONE', *, *, #783, .T. ) ;
#15084=ORIENTED_EDGE ( 'NONE', *, *, #6393, .F. ) ;
#15087=AXIS2_PLACEMENT_3D ( 'NONE', #7808, #12315, #2034 ) ;
#15089=ORIENTED_EDGE ( 'NONE', *, *, #15623, .T. ) ;
#15092=EDGE_LOOP ( 'NONE', ( #18356, #11818, #4580, #7419 ) ) ;
#15097=CARTESIAN_POINT ( 'NONE',  ( -0.9996874511566050669, -39.97499999999999432, -9.000000000000000000 ) ) ;
#15111=ORIENTED_EDGE ( 'NONE', *, *, #9442, .F. ) ;
#15116=DIRECTION ( 'NONE',  ( -0.000000000000000000, -0.000000000000000000, 1.000000000000000000 ) ) ;
#15141=DIRECTION ( 'NONE',  ( 1.000000000000000000, 0.000000000000000000, 0.000000000000000000 ) ) ;
#15146=VERTEX_POINT ( 'NONE', #13701 ) ;
#15148=ORIENTED_EDGE ( 'NONE', *, *, #5317, .T. ) ;
#15149=EDGE_CURVE ( 'NONE', #19012, #660, #6850, .T. ) ;
#15153=DIRECTION ( 'NONE',  ( 0.000000000000000000, 0.000000000000000000, 1.000000000000000000 ) ) ;
#15156=ORIENTED_EDGE ( 'NONE', *, *, #6281, .T. ) ;
#15169=CARTESIAN_POINT ( 'NONE',  ( -18.02113032590304442, -26.18033988749903074, -9.000000000000000000 ) ) ;
#15172=EDGE_LOOP ( 'NONE', ( #13370, #5186, #7088, #11968 ) ) ;
#15177=ORIENTED_EDGE ( 'NONE', *, *, #17189, .F. ) ;
#15178=DIRECTION ( 'NONE',  ( 1.000000000000000000, 0.000000000000000000, 0.000000000000000000 ) ) ;
#15184=LINE ( 'NONE', #3427, #16514 ) ;
#15186=AXIS2_PLACEMENT_3D ( 'NONE', #18727, #5465, #9781 ) ;
#15189=DIRECTION ( 'NONE',  ( 0.000000000000000000, 0.000000000000000000, 1.000000000000000000 ) ) ;
#15195=ORIENTED_EDGE ( 'NONE', *, *, #10705, .F. ) ;
#15196=DIRECTION ( 'NONE',  ( 1.000000000000000000, -6.938893903907227392E-16, 0.000000000000000000 ) ) ;
#15198=DIRECTION ( 'NONE',  ( 1.000000000000000000, 0.000000000000000000, 0.000000000000000000 ) ) ;
#15209=LINE ( 'NONE', #5105, #13898 ) ;
#15210=CARTESIAN_POINT ( 'NONE',  ( 17.79870116617236420, -10.87825472854593478, 0.000000000000000000 ) ) ;
#15218=AXIS2_PLACEMENT_3D ( 'NONE', #2545, #19215, #11526 ) ;
#15228=CARTESIAN_POINT ( 'NONE',  ( -10.93224627749298783, -36.74771600333134103, 9.000000000000000000 ) ) ;
#15258=ADVANCED_FACE ( 'NONE', ( #15271 ), #12517, .F. ) ;
#15260=ADVANCED_FACE ( 'NONE', ( #4795 ), #17046, .F. ) ;
#15266=DIRECTION ( 'NONE',  ( 0.000000000000000000, 0.000000000000000000, 1.000000000000000000 ) ) ;
#15268=AXIS2_PLACEMENT_3D ( 'NONE', #14604, #19160, #11669 ) ;
#15271=FACE_OUTER_BOUND ( 'NONE', #2468, .T. ) ;
#15282=EDGE_CURVE ( 'NONE', #6580, #6930, #17141, .T. ) ;
#15285=AXIS2_PLACEMENT_3D ( 'NONE', #18161, #3251, #9211 ) ;
#15288=DIRECTION ( 'NONE',  ( 1.000000000000000000, 0.000000000000000000, 0.000000000000000000 ) ) ;
#15292=CARTESIAN_POINT ( 'NONE',  ( 2.449293598294706513E-15, -20.00000000000000000, -8.999999999999998224 ) ) ;
#15298=LINE ( 'NONE', #13824, #3306 ) ;
#15312=VECTOR ( 'NONE', #1030, 1000.000000000000000 ) ;
#15316=ADVANCED_FACE ( 'NONE', ( #15856 ), #8293, .T. ) ;
#15330=DIRECTION ( 'NONE',  ( 0.000000000000000000, 0.000000000000000000, 1.000000000000000000 ) ) ;
#15332=CIRCLE ( 'NONE', #11878, 20.00000000000000000 ) ;
#15338=VERTEX_POINT ( 'NONE', #5161 ) ;
#15340=DIRECTION ( 'NONE',  ( 0.000000000000000000, 0.000000000000000000, 1.000000000000000000 ) ) ;
#15345=DIRECTION ( 'NONE',  ( 0.000000000000000000, 0.000000000000000000, 1.000000000000000000 ) ) ;
#15347=ORIENTED_EDGE ( 'NONE', *, *, #12145, .F. ) ;
#15357=CIRCLE ( 'NONE', #18493, 20.00000000000000000 ) ;
#15364=DIRECTION ( 'NONE',  ( -0.000000000000000000, 0.000000000000000000, -1.000000000000000000 ) ) ;
#15365=AXIS2_PLACEMENT_3D ( 'NONE', #5585, #7254, #11555 ) ;
#15367=DIRECTION ( 'NONE',  ( 1.000000000000000000, 0.000000000000000000, 0.000000000000000000 ) ) ;
#15368=AXIS2_PLACEMENT_3D ( 'NONE', #7712, #376, #7907 ) ;
#15382=CARTESIAN_POINT ( 'NONE',  ( -19.89043790736545603, -22.09056926535314602, -9.000000000000000000 ) ) ;
#15383=DIRECTION ( 'NONE',  ( 0.8090169943749464521, 0.5877852522924744694, 0.000000000000000000 ) ) ;
#15388=VERTEX_POINT ( 'NONE', #6827 ) ;
#15392=ORIENTED_EDGE ( 'NONE', *, *, #11347, .F. ) ;
#15395=ORIENTED_EDGE ( 'NONE', *, *, #14434, .T. ) ;
#15397=CARTESIAN_POINT ( 'NONE',  ( 19.76107906696387673, -16.91783288752826664, 9.000000000000000000 ) ) ;
#15406=FACE_OUTER_BOUND ( 'NONE', #19217, .T. ) ;
#15412=ORIENTED_EDGE ( 'NONE', *, *, #15149, .T. ) ;
#15422=CARTESIAN_POINT ( 'NONE',  ( 14.17539641854931176, -34.10879641843979471, -9.000000000000000000 ) ) ;
#15426=DIRECTION ( 'NONE',  ( 0.000000000000000000, 0.000000000000000000, 1.000000000000000000 ) ) ;
#15431=FACE_OUTER_BOUND ( 'NONE', #12935, .T. ) ;
#15434=ORIENTED_EDGE ( 'NONE', *, *, #5327, .F. ) ;
#15435=DIRECTION ( 'NONE',  ( 0.8090169943749546677, -0.5877852522924632561, 0.000000000000000000 ) ) ;
#15438=VERTEX_POINT ( 'NONE', #19410 ) ;
#15444=EDGE_LOOP ( 'NONE', ( #16437, #1039, #18738, #15395 ) ) ;
#15447=EDGE_CURVE ( 'NONE', #1055, #6799, #18014, .T. ) ;
#15455=ORIENTED_EDGE ( 'NONE', *, *, #19396, .T. ) ;
#15458=AXIS2_PLACEMENT_3D ( 'NONE', #10617, #19292, #13372 ) ;
#15480=CARTESIAN_POINT ( 'NONE',  ( -19.99999999999999645, -20.00000000000000000, 9.000000000000000000 ) ) ;
#15483=DIRECTION ( 'NONE',  ( 0.000000000000000000, 0.000000000000000000, 1.000000000000000000 ) ) ;
#15484=EDGE_CURVE ( 'NONE', #15338, #11405, #4037, .T. ) ;
#15486=VERTEX_POINT ( 'NONE', #19308 ) ;
#15489=CARTESIAN_POINT ( 'NONE',  ( -11.75570504584937481, -36.18033988749900942, -9.000000000000000000 ) ) ;
#15493=EDGE_CURVE ( 'NONE', #19111, #3032, #1858, .T. ) ;
#15507=AXIS2_PLACEMENT_3D ( 'NONE', #10296, #2591, #16299 ) ;
#15515=ORIENTED_EDGE ( 'NONE', *, *, #9197, .T. ) ;
#15516=LINE ( 'NONE', #9619, #8025 ) ;
#15517=CARTESIAN_POINT ( 'NONE',  ( -0.9996874511566241628, -0.02500000000000071609, -9.000000000000000000 ) ) ;
#15518=EDGE_CURVE ( 'NONE', #337, #11744, #15632, .T. ) ;
#15524=AXIS2_PLACEMENT_3D ( 'NONE', #18243, #4797, #10760 ) ;
#15553=VERTEX_POINT ( 'NONE', #15061 ) ;
#15583=CARTESIAN_POINT ( 'NONE',  ( 2.449293598294706513E-15, -20.00000000000000000, 9.000000000000000000 ) ) ;
#15602=CIRCLE ( 'NONE', #10277, 1.000000000000000888 ) ;
#15606=DIRECTION ( 'NONE',  ( -0.000000000000000000, -0.000000000000000000, -1.000000000000000000 ) ) ;
#15616=AXIS2_PLACEMENT_3D ( 'NONE', #14654, #2635, #11620 ) ;
#15623=EDGE_CURVE ( 'NONE', #8364, #18559, #8106, .T. ) ;
#15625=CARTESIAN_POINT ( 'NONE',  ( 14.86289650954800479, -33.38261212717704041, -9.000000000000000000 ) ) ;
#15632=CIRCLE ( 'NONE', #9670, 20.00000000000000000 ) ;
#15643=CARTESIAN_POINT ( 'NONE',  ( -7.134732861516020819, -1.729090847147989773, -9.000000000000000000 ) ) ;
#15656=VECTOR ( 'NONE', #11329, 1000.000000000000000 ) ;
#15657=ORIENTED_EDGE ( 'NONE', *, *, #14214, .F. ) ;
#15663=CARTESIAN_POINT ( 'NONE',  ( -14.86289650954781649, -33.38261212717723936, 9.000000000000000000 ) ) ;
#15666=VECTOR ( 'NONE', #12727, 1000.000000000000000 ) ;
#15681=CIRCLE ( 'NONE', #17577, 0.9999999999999995559 ) ;
#15688=ORIENTED_EDGE ( 'NONE', *, *, #2466, .T. ) ;
#15692=CIRCLE ( 'NONE', #13182, 20.00000000000000000 ) ;
#15729=DIRECTION ( 'NONE',  ( 0.000000000000000000, 0.000000000000000000, 1.000000000000000000 ) ) ;
#15740=ORIENTED_EDGE ( 'NONE', *, *, #16491, .F. ) ;
#15754=CYLINDRICAL_SURFACE ( 'NONE', #19140, 0.9999999999999991118 ) ;
#15756=EDGE_CURVE ( 'NONE', #2874, #6953, #13673, .T. ) ;
#15758=ORIENTED_EDGE ( 'NONE', *, *, #7587, .T. ) ;
#15805=DIRECTION ( 'NONE',  ( 0.4999999999999974465, 0.8660254037844401509, 0.000000000000000000 ) ) ;
#15806=EDGE_CURVE ( 'NONE', #17098, #3997, #925, .T. ) ;
#15815=DIRECTION ( 'NONE',  ( 1.000000000000000000, 0.000000000000000000, 0.000000000000000000 ) ) ;
#15841=CARTESIAN_POINT ( 'NONE',  ( 2.449293598294706513E-15, -20.00000000000000000, 9.000000000000000000 ) ) ;
#15844=CIRCLE ( 'NONE', #13026, 20.00000000000000000 ) ;
#15848=ORIENTED_EDGE ( 'NONE', *, *, #9867, .T. ) ;
#15852=ORIENTED_EDGE ( 'NONE', *, *, #8813, .F. ) ;
#15856=FACE_OUTER_BOUND ( 'NONE', #2869, .T. ) ;
#15861=VERTEX_POINT ( 'NONE', #3775 ) ;
#15865=DIRECTION ( 'NONE',  ( 0.000000000000000000, -0.000000000000000000, 1.000000000000000000 ) ) ;
#15867=AXIS2_PLACEMENT_3D ( 'NONE', #15041, #16623, #9237 ) ;
#15870=CARTESIAN_POINT ( 'NONE',  ( -3.158233816355059620, -39.56295201467614220, -9.000000000000000000 ) ) ;
#15874=ORIENTED_EDGE ( 'NONE', *, *, #11792, .T. ) ;
#15884=ORIENTED_EDGE ( 'NONE', *, *, #4788, .T. ) ;
#15903=FACE_OUTER_BOUND ( 'NONE', #826, .T. ) ;
#15917=( LENGTH_UNIT ( ) NAMED_UNIT ( * ) SI_UNIT ( .MILLI., .METRE. ) );
#15921=CIRCLE ( 'NONE', #6216, 5.000000000000000888 ) ;
#15922=DIRECTION ( 'NONE',  ( -0.000000000000000000, 0.000000000000000000, 1.000000000000000000 ) ) ;
#15923=DIRECTION ( 'NONE',  ( 1.000000000000000000, 0.000000000000000000, 0.000000000000000000 ) ) ;
#15924=ORIENTED_EDGE ( 'NONE', *, *, #15518, .F. ) ;
#15947=VERTEX_POINT ( 'NONE', #2615 ) ;
#15949=VERTEX_POINT ( 'NONE', #11599 ) ;
#15955=DIRECTION ( 'NONE',  ( -1.000000000000000000, 0.000000000000000000, 0.000000000000000000 ) ) ;
#15957=ORIENTED_EDGE ( 'NONE', *, *, #2382, .T. ) ;
#15961=CARTESIAN_POINT ( 'NONE',  ( -4.158233816355195955, -0.4370479853238878887, -9.000000000000000000 ) ) ;
#15964=AXIS2_PLACEMENT_3D ( 'NONE', #15583, #5095, #18555 ) ;
#15970=AXIS2_PLACEMENT_3D ( 'NONE', #11184, #8343, #6781 ) ;
#16014=DIRECTION ( 'NONE',  ( 1.000000000000000000, 0.000000000000000000, 0.000000000000000000 ) ) ;
#16031=CARTESIAN_POINT ( 'NONE',  ( 2.449293598294706513E-15, -20.00000000000000000, 9.000000000000000000 ) ) ;
#16032=EDGE_LOOP ( 'NONE', ( #5092, #12810, #2551, #1072, #14197, #17021, #1844, #18401, #727, #13058, #3646, #5796, #10851, #3668, #1077, #7974, #4488, #17488, #8903, #4945, #9745, #13217, #6413, #9643, #13155, #10128, #8861, #8179, #3290, #11454, #15740, #11520, #12956, #1280, #17951, #5113, #6258, #10354, #16472, #11842, #13311, #11104, #17025, #8242, #5387, #922, #2729, #14350, #11306, #14246, #179, #9618, #7113, #388, #4889, #18937, #15434, #14249, #1456, #17408, #13121, #7406, #2924, #15054, #15412, #9633, #13132, #9733, #5947, #10681, #19257, #2612, #6028, #17613, #13608 ) ) ;
#16033=DIRECTION ( 'NONE',  ( 0.000000000000000000, 0.000000000000000000, 1.000000000000000000 ) ) ;
#16042=EDGE_CURVE ( 'NONE', #11631, #17511, #4979, .T. ) ;
#16049=DIRECTION ( 'NONE',  ( 0.000000000000000000, 0.000000000000000000, 1.000000000000000000 ) ) ;
#16051=AXIS2_PLACEMENT_3D ( 'NONE', #17806, #4661, #7781 ) ;
#16052=ORIENTED_EDGE ( 'NONE', *, *, #15282, .F. ) ;
#16065=ORIENTED_EDGE ( 'NONE', *, *, #892, .T. ) ;
#16068=DIRECTION ( 'NONE',  ( -1.000000000000000000, 0.000000000000000000, 0.000000000000000000 ) ) ;
#16083=ORIENTED_EDGE ( 'NONE', *, *, #10462, .T. ) ;
#16088=LINE ( 'NONE', #1086, #13605 ) ;
#16103=CARTESIAN_POINT ( 'NONE',  ( 7.211304515372821022, -38.65468003441933575, 0.000000000000000000 ) ) ;
#16115=CARTESIAN_POINT ( 'NONE',  ( -17.32050807568872841, -30.00000000000008171, -9.000000000000000000 ) ) ;
#16137=CARTESIAN_POINT ( 'NONE',  ( -14.17539641854911459, -34.10879641843998655, 9.000000000000000000 ) ) ;
#16140=CARTESIAN_POINT ( 'NONE',  ( 2.449293598294706513E-15, -20.00000000000000000, -9.000000000000000000 ) ) ;
#16143=CIRCLE ( 'NONE', #1101, 0.9999999999999991118 ) ;
#16155=DIRECTION ( 'NONE',  ( 0.000000000000000000, 0.000000000000000000, 1.000000000000000000 ) ) ;
#16161=DIRECTION ( 'NONE',  ( 1.000000000000000000, 0.000000000000000000, 0.000000000000000000 ) ) ;
#16171=VERTEX_POINT ( 'NONE', #9231 ) ;
#16175=EDGE_LOOP ( 'NONE', ( #8409, #8965, #8052, #12015 ) ) ;
#16183=CARTESIAN_POINT ( 'NONE',  ( -14.86289650954790886, -6.617387872822862782, -9.000000000000000000 ) ) ;
#16189=AXIS2_PLACEMENT_3D ( 'NONE', #13932, #9332, #513 ) ;
#16190=DIRECTION ( 'NONE',  ( 0.000000000000000000, 0.000000000000000000, 1.000000000000000000 ) ) ;
#16191=DIRECTION ( 'NONE',  ( 1.000000000000000000, 0.000000000000000000, 0.000000000000000000 ) ) ;
#16192=AXIS2_PLACEMENT_3D ( 'NONE', #716, #3753, #9719 ) ;
#16196=DIRECTION ( 'NONE',  ( -0.000000000000000000, 0.000000000000000000, 1.000000000000000000 ) ) ;
#16201=DIRECTION ( 'NONE',  ( 0.000000000000000000, 0.000000000000000000, 1.000000000000000000 ) ) ;
#16207=DIRECTION ( 'NONE',  ( 0.000000000000000000, -0.000000000000000000, 1.000000000000000000 ) ) ;
#16215=VERTEX_POINT ( 'NONE', #6309 ) ;
#16218=ORIENTED_EDGE ( 'NONE', *, *, #9868, .T. ) ;
#16219=CARTESIAN_POINT ( 'NONE',  ( -4.158233816355060064, -39.56295201467614220, -9.000000000000000000 ) ) ;
#16240=ADVANCED_FACE ( 'NONE', ( #12951 ), #5207, .T. ) ;
#16241=ORIENTED_EDGE ( 'NONE', *, *, #17684, .T. ) ;
#16246=CARTESIAN_POINT ( 'NONE',  ( 4.158233816354936607, -0.4370479853238358192, -9.000000000000000000 ) ) ;
#16275=DIRECTION ( 'NONE',  ( 0.000000000000000000, 0.000000000000000000, 1.000000000000000000 ) ) ;
#16281=CYLINDRICAL_SURFACE ( 'NONE', #5989, 1.000000000000000888 ) ;
#16297=AXIS2_PLACEMENT_3D ( 'NONE', #5941, #10335, #16339 ) ;
#16299=DIRECTION ( 'NONE',  ( -1.000000000000000000, 0.000000000000000000, 0.000000000000000000 ) ) ;
#16308=CIRCLE ( 'NONE', #7838, 20.00000000000000000 ) ;
#16318=ORIENTED_EDGE ( 'NONE', *, *, #3904, .T. ) ;
#16321=ORIENTED_EDGE ( 'NONE', *, *, #18752, .T. ) ;
#16323=CIRCLE ( 'NONE', #6917, 20.00000000000000000 ) ;
#16338=DIRECTION ( 'NONE',  ( 0.000000000000000000, 0.000000000000000000, 1.000000000000000000 ) ) ;
#16339=DIRECTION ( 'NONE',  ( 1.000000000000000000, 0.000000000000000000, 0.000000000000000000 ) ) ;
#16340=VERTEX_POINT ( 'NONE', #18866 ) ;
#16357=CARTESIAN_POINT ( 'NONE',  ( 2.449293598294706513E-15, -20.00000000000000000, -9.000000000000000000 ) ) ;
#16363=CYLINDRICAL_SURFACE ( 'NONE', #18344, 1.000000000000000888 ) ;
#16372=EDGE_CURVE ( 'NONE', #7491, #439, #7464, .T. ) ;
#16376=VERTEX_POINT ( 'NONE', #8737 ) ;
#16387=DIRECTION ( 'NONE',  ( -0.000000000000000000, -0.000000000000000000, -1.000000000000000000 ) ) ;
#16400=DIRECTION ( 'NONE',  ( 0.1045284632676635322, -0.9945218953682722907, 0.000000000000000000 ) ) ;
#16404=DIRECTION ( 'NONE',  ( 1.000000000000000000, 0.000000000000000000, 0.000000000000000000 ) ) ;
#16407=DIRECTION ( 'NONE',  ( 1.000000000000000000, 0.000000000000000000, 0.000000000000000000 ) ) ;
#16415=AXIS2_PLACEMENT_3D ( 'NONE', #8865, #10325, #6214 ) ;
#16423=ORIENTED_EDGE ( 'NONE', *, *, #11327, .T. ) ;
#16437=ORIENTED_EDGE ( 'NONE', *, *, #10875, .F. ) ;
#16440=VERTEX_POINT ( 'NONE', #14515 ) ;
#16443=ORIENTED_EDGE ( 'NONE', *, *, #5168, .T. ) ;
#16444=CIRCLE ( 'NONE', #17382, 0.9999999999999997780 ) ;
#16452=AXIS2_PLACEMENT_3D ( 'NONE', #11761, #19165, #1196 ) ;
#16462=ORIENTED_EDGE ( 'NONE', *, *, #4020, .F. ) ;
#16472=ORIENTED_EDGE ( 'NONE', *, *, #14578, .F. ) ;
#16479=VECTOR ( 'NONE', #10948, 1000.000000000000000 ) ;
#16480=EDGE_CURVE ( 'NONE', #14983, #8685, #9061, .T. ) ;
#16482=EDGE_CURVE ( 'NONE', #10947, #4767, #13248, .T. ) ;
#16487=FACE_OUTER_BOUND ( 'NONE', #14730, .T. ) ;
#16491=EDGE_CURVE ( 'NONE', #11186, #1055, #6873, .T. ) ;
#16494=ORIENTED_EDGE ( 'NONE', *, *, #17259, .F. ) ;
#16497=CARTESIAN_POINT ( 'NONE',  ( 19.30627432446651781, -25.22185519795838715, -9.000000000000000000 ) ) ;
#16504=CIRCLE ( 'NONE', #16192, 1.000000000000000222 ) ;
#16514=VECTOR ( 'NONE', #6172, 1000.000000000000000 ) ;
#16520=VERTEX_POINT ( 'NONE', #5603 ) ;
#16531=DIRECTION ( 'NONE',  ( -0.1045284632676425907, -0.9945218953682745111, 0.000000000000000000 ) ) ;
#16540=ORIENTED_EDGE ( 'NONE', *, *, #4256, .F. ) ;
#16543=ADVANCED_FACE ( 'NONE', ( #7272 ), #17588, .T. ) ;
#16545=ORIENTED_EDGE ( 'NONE', *, *, #9721, .T. ) ;
#16547=EDGE_LOOP ( 'NONE', ( #15848, #14683, #4771, #47 ) ) ;
#16560=VERTEX_POINT ( 'NONE', #8638 ) ;
#16569=VERTEX_POINT ( 'NONE', #16497 ) ;
#16571=VECTOR ( 'NONE', #17817, 1000.000000000000000 ) ;
#16576=DIRECTION ( 'NONE',  ( -0.000000000000000000, -0.000000000000000000, -1.000000000000000000 ) ) ;
#16577=DIRECTION ( 'NONE',  ( 0.6691306063588571273, 0.7431448254773952433, 0.000000000000000000 ) ) ;
#16583=ORIENTED_EDGE ( 'NONE', *, *, #2247, .T. ) ;
#16587=VECTOR ( 'NONE', #11813, 1000.000000000000000 ) ;
#16610=VERTEX_POINT ( 'NONE', #15397 ) ;
#16611=VECTOR ( 'NONE', #11158, 1000.000000000000000 ) ;
#16613=EDGE_CURVE ( 'NONE', #17604, #6538, #2532, .T. ) ;
#16617=ORIENTED_EDGE ( 'NONE', *, *, #15006, .F. ) ;
#16622=ORIENTED_EDGE ( 'NONE', *, *, #13945, .F. ) ;
#16623=DIRECTION ( 'NONE',  ( 0.000000000000000000, -0.000000000000000000, 1.000000000000000000 ) ) ;
#16624=FACE_OUTER_BOUND ( 'NONE', #16032, .T. ) ;
#16627=DIRECTION ( 'NONE',  ( -0.000000000000000000, -0.000000000000000000, -1.000000000000000000 ) ) ;
#16638=DIRECTION ( 'NONE',  ( -0.000000000000000000, -0.000000000000000000, 1.000000000000000000 ) ) ;
#16646=ORIENTED_EDGE ( 'NONE', *, *, #14789, .T. ) ;
#16670=CARTESIAN_POINT ( 'NONE',  ( 2.449293598294706513E-15, -20.00000000000000000, 9.000000000000000000 ) ) ;
#16686=CARTESIAN_POINT ( 'NONE',  ( 2.449293598294706513E-15, -20.00000000000000000, -9.000000000000000000 ) ) ;
#16691=DIRECTION ( 'NONE',  ( 1.000000000000000000, 0.000000000000000000, 0.000000000000000000 ) ) ;
#16702=CARTESIAN_POINT ( 'NONE',  ( 2.449293598294706513E-15, -20.00000000000000000, 9.000000000000000000 ) ) ;
#16713=CARTESIAN_POINT ( 'NONE',  ( 9.037824375505316254, -2.158539001597377105, 0.000000000000000000 ) ) ;
#16722=EDGE_CURVE ( 'NONE', #5652, #8510, #625, .T. ) ;
#16725=AXIS2_PLACEMENT_3D ( 'NONE', #914, #19176, #7378 ) ;
#16732=EDGE_CURVE ( 'NONE', #6328, #13819, #1269, .T. ) ;
#16739=EDGE_LOOP ( 'NONE', ( #10581, #17030, #1777, #9497 ) ) ;
#16741=DIRECTION ( 'NONE',  ( 0.000000000000000000, 0.000000000000000000, 1.000000000000000000 ) ) ;
#16748=CARTESIAN_POINT ( 'NONE',  ( -7.211304515372548352, -38.65468003441944944, -9.000000000000000000 ) ) ;
#16757=CIRCLE ( 'NONE', #16452, 1.000000000000000222 ) ;
#16768=LINE ( 'NONE', #18250, #17074 ) ;
#16772=DIRECTION ( 'NONE',  ( 0.000000000000000000, 0.000000000000000000, 1.000000000000000000 ) ) ;
#16776=CARTESIAN_POINT ( 'NONE',  ( 2.449293598294706513E-15, -20.00000000000000000, 9.000000000000000000 ) ) ;
#16783=DIRECTION ( 'NONE',  ( 0.000000000000000000, 0.000000000000000000, 1.000000000000000000 ) ) ;
#16789=CIRCLE ( 'NONE', #19000, 1.000000000000001110 ) ;
#16796=AXIS2_PLACEMENT_3D ( 'NONE', #6933, #12913, #14479 ) ;
#16798=ORIENTED_EDGE ( 'NONE', *, *, #7237, .T. ) ;
#16805=ORIENTED_EDGE ( 'NONE', *, *, #7636, .T. ) ;
#16811=CYLINDRICAL_SURFACE ( 'NONE', #2686, 20.00000000000000000 ) ;
#16826=CARTESIAN_POINT ( 'NONE',  ( 2.449293598294706513E-15, -20.00000000000000000, 9.000000000000000000 ) ) ;
#16830=EDGE_CURVE ( 'NONE', #19111, #5570, #3726, .T. ) ;
#16833=ORIENTED_EDGE ( 'NONE', *, *, #13526, .T. ) ;
#16856=CIRCLE ( 'NONE', #4319, 20.00000000000000000 ) ;
#16859=EDGE_CURVE ( 'NONE', #8337, #10629, #3538, .T. ) ;
#16862=ORIENTED_EDGE ( 'NONE', *, *, #18497, .T. ) ;
#16864=FACE_OUTER_BOUND ( 'NONE', #19030, .T. ) ;
#16867=VECTOR ( 'NONE', #13312, 1000.000000000000000 ) ;
#16895=CIRCLE ( 'NONE', #15007, 20.00000000000000000 ) ;
#16898=ADVANCED_FACE ( 'NONE', ( #8127 ), #18737, .F. ) ;
#16906=CARTESIAN_POINT ( 'NONE',  ( -19.02113032590308705, -13.81966011250110249, -9.000000000000000000 ) ) ;
#16908=CARTESIAN_POINT ( 'NONE',  ( 10.93224627749286526, -3.252283996668575483, -9.000000000000000000 ) ) ;
#16911=CARTESIAN_POINT ( 'NONE',  ( -5.130877905917148318, -39.33065161639853358, 9.000000000000000000 ) ) ;
#16912=VECTOR ( 'NONE', #8538, 1000.000000000000000 ) ;
#16933=DIRECTION ( 'NONE',  ( 1.000000000000000000, 0.000000000000000000, 0.000000000000000000 ) ) ;
#16949=AXIS2_PLACEMENT_3D ( 'NONE', #882, #14007, #18560 ) ;
#16955=AXIS2_PLACEMENT_3D ( 'NONE', #15625, #15922, #2507 ) ;
#16960=CARTESIAN_POINT ( 'NONE',  ( 4.158233816355333623, -39.56295201467608535, 9.000000000000000000 ) ) ;
#16972=EDGE_CURVE ( 'NONE', #17065, #2854, #3463, .T. ) ;
#16976=ORIENTED_EDGE ( 'NONE', *, *, #3457, .T. ) ;
#16997=DIRECTION ( 'NONE',  ( -0.000000000000000000, -0.000000000000000000, 1.000000000000000000 ) ) ;
#17004=FACE_OUTER_BOUND ( 'NONE', #16175, .T. ) ;
#17006=LINE ( 'NONE', #811, #5843 ) ;
#17007=CARTESIAN_POINT ( 'NONE',  ( 1.000000000000000000, -14.00000000000000000, -9.000000000000001776 ) ) ;
#17020=EDGE_LOOP ( 'NONE', ( #17236, #19314, #956, #13200 ) ) ;
#17021=ORIENTED_EDGE ( 'NONE', *, *, #12145, .T. ) ;
#17023=ORIENTED_EDGE ( 'NONE', *, *, #16732, .T. ) ;
#17025=ORIENTED_EDGE ( 'NONE', *, *, #13755, .T. ) ;
#17030=ORIENTED_EDGE ( 'NONE', *, *, #6064, .F. ) ;
#17042=CARTESIAN_POINT ( 'NONE',  ( -19.02113032590304442, -26.18033988749903074, -9.000000000000000000 ) ) ;
#17046=CYLINDRICAL_SURFACE ( 'NONE', #8093, 1.000000000000000888 ) ;
#17051=ORIENTED_EDGE ( 'NONE', *, *, #9160, .T. ) ;
#17063=AXIS2_PLACEMENT_3D ( 'NONE', #9132, #5902, #11870 ) ;
#17065=VERTEX_POINT ( 'NONE', #15013 ) ;
#17071=DIRECTION ( 'NONE',  ( 1.000000000000000000, 0.000000000000000000, 0.000000000000000000 ) ) ;
#17074=VECTOR ( 'NONE', #392, 1000.000000000000000 ) ;
#17079=DIRECTION ( 'NONE',  ( 1.000000000000000000, 0.000000000000000000, 0.000000000000000000 ) ) ;
#17083=CARTESIAN_POINT ( 'NONE',  ( -12.54977455159125377, -4.427487078052159575, -9.000000000000000000 ) ) ;
#17089=EDGE_LOOP ( 'NONE', ( #2058, #17051, #19188, #13561 ) ) ;
#17094=DIRECTION ( 'NONE',  ( 1.000000000000000000, 0.000000000000000000, 0.000000000000000000 ) ) ;
#17098=VERTEX_POINT ( 'NONE', #8030 ) ;
#17103=DIRECTION ( 'NONE',  ( 0.000000000000000000, 0.000000000000000000, 1.000000000000000000 ) ) ;
#17112=DIRECTION ( 'NONE',  ( 1.000000000000000000, 0.000000000000000000, 0.000000000000000000 ) ) ;
#17124=LINE ( 'NONE', #14059, #12950 ) ;
#17125=PRODUCT_DEFINITION_SHAPE ( 'NONE', 'NONE',  #5304 ) ;
#17141=LINE ( 'NONE', #13005, #1220 ) ;
#17143=ORIENTED_EDGE ( 'NONE', *, *, #9097, .F. ) ;
#17149=LINE ( 'NONE', #4002, #19354 ) ;
#17153=DIRECTION ( 'NONE',  ( 0.000000000000000000, 0.000000000000000000, 1.000000000000000000 ) ) ;
#17156=VECTOR ( 'NONE', #2779, 1000.000000000000000 ) ;
#17160=FILL_AREA_STYLE_COLOUR ( '', #14339 ) ;
#17162=CARTESIAN_POINT ( 'NONE',  ( 2.449293598294706513E-15, -20.00000000000000000, -9.000000000000000000 ) ) ;
#17164=CARTESIAN_POINT ( 'NONE',  ( -15.51323935927264586, -32.62297130559655045, -9.000000000000000000 ) ) ;
#17165=DIRECTION ( 'NONE',  ( 0.000000000000000000, 0.000000000000000000, -1.000000000000000000 ) ) ;
#17167=AXIS2_PLACEMENT_3D ( 'NONE', #10521, #13570, #142 ) ;
#17175=MECHANICAL_DESIGN_GEOMETRIC_PRESENTATION_REPRESENTATION('',(#3103),#18443);
#17182=AXIS2_PLACEMENT_3D ( 'NONE', #18640, #3720, #9684 ) ;
#17186=EDGE_CURVE ( 'NONE', #4192, #17315, #12230, .T. ) ;
#17189=EDGE_CURVE ( 'NONE', #8857, #10940, #11161, .T. ) ;
#17197=EDGE_CURVE ( 'NONE', #15861, #13867, #3784, .T. ) ;
#17204=CARTESIAN_POINT ( 'NONE',  ( 2.449293598294706513E-15, -20.00000000000000000, -9.000000000000000000 ) ) ;
#17206=EDGE_CURVE ( 'NONE', #16376, #12683, #11278, .T. ) ;
#17212=ORIENTED_EDGE ( 'NONE', *, *, #2839, .T. ) ;
#17220=EDGE_LOOP ( 'NONE', ( #9254, #18094, #7747, #129 ) ) ;
#17227=AXIS2_PLACEMENT_3D ( 'NONE', #5898, #2877, #17677 ) ;
#17232=ORIENTED_EDGE ( 'NONE', *, *, #7935, .T. ) ;
#17236=ORIENTED_EDGE ( 'NONE', *, *, #6288, .F. ) ;
#17258=AXIS2_PLACEMENT_3D ( 'NONE', #6466, #14202, #17272 ) ;
#17259=EDGE_CURVE ( 'NONE', #16560, #10123, #19146, .T. ) ;
#17265=( NAMED_UNIT ( * ) PLANE_ANGLE_UNIT ( ) SI_UNIT ( $, .RADIAN. ) );
#17272=DIRECTION ( 'NONE',  ( 0.4999999999999974465, 0.8660254037844401509, 0.000000000000000000 ) ) ;
#17276=CARTESIAN_POINT ( 'NONE',  ( 16.79901371501595975, -30.85325472854598416, 9.000000000000000000 ) ) ;
#17279=CARTESIAN_POINT ( 'NONE',  ( -4.158233816355195955, -0.4370479853238878887, -9.000000000000000000 ) ) ;
#17294=DIRECTION ( 'NONE',  ( -1.000000000000000000, 0.000000000000000000, 0.000000000000000000 ) ) ;
#17310=DIRECTION ( 'NONE',  ( 0.000000000000000000, -0.000000000000000000, 1.000000000000000000 ) ) ;
#17311=ORIENTED_EDGE ( 'NONE', *, *, #18752, .F. ) ;
#17313=EDGE_CURVE ( 'NONE', #6336, #17942, #2471, .T. ) ;
#17315=VERTEX_POINT ( 'NONE', #9888 ) ;
#17323=ADVANCED_FACE ( 'NONE', ( #8529 ), #4120, .T. ) ;
#17331=DIRECTION ( 'NONE',  ( 0.000000000000000000, -0.000000000000000000, 1.000000000000000000 ) ) ;
#17333=EDGE_CURVE ( 'NONE', #16171, #666, #1913, .T. ) ;
#17347=ORIENTED_EDGE ( 'NONE', *, *, #6851, .T. ) ;
#17350=FACE_OUTER_BOUND ( 'NONE', #7725, .T. ) ;
#17360=CARTESIAN_POINT ( 'NONE',  ( 2.449293598294706513E-15, -20.00000000000000000, 9.000000000000000000 ) ) ;
#17368=DIRECTION ( 'NONE',  ( 0.000000000000000000, 0.000000000000000000, 1.000000000000000000 ) ) ;
#17373=DIRECTION ( 'NONE',  ( 1.000000000000000000, 0.000000000000000000, 0.000000000000000000 ) ) ;
#17382=AXIS2_PLACEMENT_3D ( 'NONE', #14994, #17960, #4314 ) ;
#17398=CIRCLE ( 'NONE', #12650, 0.9999999999999995559 ) ;
#17401=CARTESIAN_POINT ( 'NONE',  ( -1.000000000000000000, -14.00000000000000000, 8.999999999999998224 ) ) ;
#17408=ORIENTED_EDGE ( 'NONE', *, *, #281, .F. ) ;
#17424=LINE ( 'NONE', #9760, #15656 ) ;
#17430=ADVANCED_FACE ( 'NONE', ( #7344 ), #13320, .F. ) ;
#17435=ORIENTED_EDGE ( 'NONE', *, *, #9632, .F. ) ;
#17449=CARTESIAN_POINT ( 'NONE',  ( 16.79901371501573593, -9.146745271453662340, 9.000000000000000000 ) ) ;
#17451=ORIENTED_EDGE ( 'NONE', *, *, #6870, .T. ) ;
#17454=EDGE_CURVE ( 'NONE', #5652, #11251, #3478, .T. ) ;
#17455=AXIS2_PLACEMENT_3D ( 'NONE', #16906, #18580, #6485 ) ;
#17464=CARTESIAN_POINT ( 'NONE',  ( 16.79901371501573593, -9.146745271453662340, 0.000000000000000000 ) ) ;
#17479=ADVANCED_FACE ( 'NONE', ( #11847 ), #16281, .F. ) ;
#17484=DIRECTION ( 'NONE',  ( -1.000000000000000000, 0.000000000000000000, 0.000000000000000000 ) ) ;
#17488=ORIENTED_EDGE ( 'NONE', *, *, #934, .T. ) ;
#17489=FACE_OUTER_BOUND ( 'NONE', #2308, .T. ) ;
#17497=AXIS2_PLACEMENT_3D ( 'NONE', #16776, #7840, #13023 ) ;
#17500=ORIENTED_EDGE ( 'NONE', *, *, #5669, .F. ) ;
#17511=VERTEX_POINT ( 'NONE', #193 ) ;
#17515=CARTESIAN_POINT ( 'NONE',  ( 2.449293598294706513E-15, -20.00000000000000000, 9.000000000000000000 ) ) ;
#17534=ORIENTED_EDGE ( 'NONE', *, *, #14633, .T. ) ;
#17546=DIRECTION ( 'NONE',  ( 0.000000000000000000, 0.000000000000000000, 1.000000000000000000 ) ) ;
#17548=DIRECTION ( 'NONE',  ( 0.000000000000000000, 0.000000000000000000, 1.000000000000000000 ) ) ;
#17552=FACE_OUTER_BOUND ( 'NONE', #11554, .T. ) ;
#17558=AXIS2_PLACEMENT_3D ( 'NONE', #16826, #15345, #1928 ) ;
#17570=CYLINDRICAL_SURFACE ( 'NONE', #10475, 20.00000000000000000 ) ;
#17577=AXIS2_PLACEMENT_3D ( 'NONE', #7580, #17898, #13269 ) ;
#17582=CYLINDRICAL_SURFACE ( 'NONE', #5260, 1.000000000000000000 ) ;
#17588=CYLINDRICAL_SURFACE ( 'NONE', #9378, 20.00000000000000000 ) ;
#17604=VERTEX_POINT ( 'NONE', #10764 ) ;
#17605=MECHANICAL_DESIGN_GEOMETRIC_PRESENTATION_REPRESENTATION('',(#1940),#18240);
#17610=ORIENTED_EDGE ( 'NONE', *, *, #18164, .F. ) ;
#17611=CARTESIAN_POINT ( 'NONE',  ( -14.86289650954790886, -6.617387872822862782, -9.000000000000000000 ) ) ;
#17613=ORIENTED_EDGE ( 'NONE', *, *, #4959, .T. ) ;
#17630=ORIENTED_EDGE ( 'NONE', *, *, #10462, .F. ) ;
#17631=CARTESIAN_POINT ( 'NONE',  ( -3.175194142252219631, -0.2536549670829672531, 0.000000000000000000 ) ) ;
#17635=DIRECTION ( 'NONE',  ( 0.000000000000000000, 0.000000000000000000, 1.000000000000000000 ) ) ;
#17640=ORIENTED_EDGE ( 'NONE', *, *, #9632, .T. ) ;
#17645=DIRECTION ( 'NONE',  ( -0.000000000000000000, -0.000000000000000000, -1.000000000000000000 ) ) ;
#17650=ORIENTED_EDGE ( 'NONE', *, *, #9630, .F. ) ;
#17659=DIRECTION ( 'NONE',  ( 0.000000000000000000, 0.000000000000000000, -1.000000000000000000 ) ) ;
#17677=DIRECTION ( 'NONE',  ( 1.000000000000000000, 0.000000000000000000, 0.000000000000000000 ) ) ;
#17679=EDGE_CURVE ( 'NONE', #15861, #10123, #15692, .T. ) ;
#17684=EDGE_CURVE ( 'NONE', #5943, #508, #18628, .T. ) ;
#17707=DIRECTION ( 'NONE',  ( -0.000000000000000000, -0.000000000000000000, -1.000000000000000000 ) ) ;
#17716=VERTEX_POINT ( 'NONE', #4981 ) ;
#17718=DIRECTION ( 'NONE',  ( 1.000000000000000000, 0.000000000000000000, 0.000000000000000000 ) ) ;
#17731=VERTEX_POINT ( 'NONE', #4837 ) ;
#17732=DIRECTION ( 'NONE',  ( -0.000000000000000000, -0.000000000000000000, 1.000000000000000000 ) ) ;
#17739=EDGE_CURVE ( 'NONE', #3362, #1643, #19164, .T. ) ;
#17754=CARTESIAN_POINT ( 'NONE',  ( 17.79870116617256315, -29.12174527145368330, -9.000000000000000000 ) ) ;
#17770=CARTESIAN_POINT ( 'NONE',  ( 2.449293598294706513E-15, -20.00000000000000000, -9.000000000000000000 ) ) ;
#17771=CIRCLE ( 'NONE', #13683, 20.00000000000000000 ) ;
#17790=DIRECTION ( 'NONE',  ( 1.000000000000000000, 0.000000000000000000, 0.000000000000000000 ) ) ;
#17797=CYLINDRICAL_SURFACE ( 'NONE', #11282, 0.9999999999999991118 ) ;
#17798=EDGE_CURVE ( 'NONE', #14027, #3339, #15332, .T. ) ;
#17801=ORIENTED_EDGE ( 'NONE', *, *, #6332, .F. ) ;
#17806=CARTESIAN_POINT ( 'NONE',  ( 17.32050807568866091, -9.999999999999797495, -9.000000000000000000 ) ) ;
#17812=EDGE_CURVE ( 'NONE', #3235, #3752, #4381, .T. ) ;
#17814=DIRECTION ( 'NONE',  ( -1.000000000000000000, 0.000000000000000000, 0.000000000000000000 ) ) ;
#17817=DIRECTION ( 'NONE',  ( -0.000000000000000000, -0.000000000000000000, 1.000000000000000000 ) ) ;
#17818=ORIENTED_EDGE ( 'NONE', *, *, #8553, .T. ) ;
#17822=DIRECTION ( 'NONE',  ( 0.000000000000000000, 0.000000000000000000, 1.000000000000000000 ) ) ;
#17827=FACE_OUTER_BOUND ( 'NONE', #13196, .T. ) ;
#17845=DIRECTION ( 'NONE',  ( 1.000000000000000000, 0.000000000000000000, 0.000000000000000000 ) ) ;
#17846=EDGE_LOOP ( 'NONE', ( #8832, #18213, #7813, #1316 ) ) ;
#17855=AXIS2_PLACEMENT_3D ( 'NONE', #8549, #14517, #18963 ) ;
#17859=DIRECTION ( 'NONE',  ( -0.1045284632676563297, 0.9945218953682731788, 0.000000000000000000 ) ) ;
#17871=CIRCLE ( 'NONE', #14397, 20.00000000000000000 ) ;
#17873=DIRECTION ( 'NONE',  ( -0.000000000000000000, -0.000000000000000000, 1.000000000000000000 ) ) ;
#17883=DIRECTION ( 'NONE',  ( -1.000000000000000000, 0.000000000000000000, 0.000000000000000000 ) ) ;
#17898=DIRECTION ( 'NONE',  ( 0.000000000000000000, 0.000000000000000000, 1.000000000000000000 ) ) ;
#17901=CARTESIAN_POINT ( 'NONE',  ( 14.17539641854900978, -5.891203581559908642, -9.000000000000000000 ) ) ;
#17902=ORIENTED_EDGE ( 'NONE', *, *, #12626, .F. ) ;
#17904=FACE_BOUND ( 'NONE', #11013, .T. ) ;
#17919=APPLICATION_CONTEXT ( 'automotive_design' ) ;
#17921=VERTEX_POINT ( 'NONE', #8248 ) ;
#17942=VERTEX_POINT ( 'NONE', #4441 ) ;
#17944=ORIENTED_EDGE ( 'NONE', *, *, #10684, .T. ) ;
#17951=ORIENTED_EDGE ( 'NONE', *, *, #4076, .F. ) ;
#17953=EDGE_LOOP ( 'NONE', ( #6232, #6206, #18398, #1360 ) ) ;
#17957=CARTESIAN_POINT ( 'NONE',  ( 8.134732861516145164, -38.27090915285195649, -9.000000000000000000 ) ) ;
#17960=DIRECTION ( 'NONE',  ( 0.000000000000000000, 0.000000000000000000, 1.000000000000000000 ) ) ;
#17969=CARTESIAN_POINT ( 'NONE',  ( -10.75570504584948139, -3.819660112501066518, -9.000000000000000000 ) ) ;
#17971=ADVANCED_FACE ( 'NONE', ( #11577 ), #12954, .T. ) ;
#17980=DIRECTION ( 'NONE',  ( 1.000000000000000000, 0.000000000000000000, 0.000000000000000000 ) ) ;
#17992=ORIENTED_EDGE ( 'NONE', *, *, #14293, .T. ) ;
#17993=DIRECTION ( 'NONE',  ( 1.000000000000000000, 0.000000000000000000, 0.000000000000000000 ) ) ;
#17998=CARTESIAN_POINT ( 'NONE',  ( 2.449293598294706513E-15, -20.00000000000000000, 9.000000000000000000 ) ) ;
#18014=LINE ( 'NONE', #10532, #12468 ) ;
#18021=VERTEX_POINT ( 'NONE', #7173 ) ;
#18035=VECTOR ( 'NONE', #13444, 1000.000000000000000 ) ;
#18040=CARTESIAN_POINT ( 'NONE',  ( 2.449293598294706513E-15, -20.00000000000000000, 9.000000000000000000 ) ) ;
#18043=CIRCLE ( 'NONE', #5180, 1.000000000000000000 ) ;
#18053=CARTESIAN_POINT ( 'NONE',  ( 2.449293598294706513E-15, -20.00000000000000000, -8.999999999999998224 ) ) ;
#18066=ORIENTED_EDGE ( 'NONE', *, *, #13692, .T. ) ;
#18068=DIRECTION ( 'NONE',  ( -0.3090169943749382919, -0.9510565162951566398, 0.000000000000000000 ) ) ;
#18072=CARTESIAN_POINT ( 'NONE',  ( -0.9999999999999995559, -15.10102051443364246, -8.999999999999998224 ) ) ;
#18082=CARTESIAN_POINT ( 'NONE',  ( 2.449293598294706513E-15, -20.00000000000000000, 9.000000000000000000 ) ) ;
#18091=CARTESIAN_POINT ( 'NONE',  ( 7.211304515372821022, -38.65468003441933575, -9.000000000000000000 ) ) ;
#18094=ORIENTED_EDGE ( 'NONE', *, *, #15282, .T. ) ;
#18096=PLANE ( 'NONE',  #15458 ) ;
#18118=CIRCLE ( 'NONE', #3378, 20.00000000000000000 ) ;
#18119=ORIENTED_EDGE ( 'NONE', *, *, #5991, .F. ) ;
#18120=LINE ( 'NONE', #13499, #13813 ) ;
#18121=ORIENTED_EDGE ( 'NONE', *, *, #5852, .T. ) ;
#18129=CARTESIAN_POINT ( 'NONE',  ( 10.93224627749321876, -36.74771600333119181, 0.000000000000000000 ) ) ;
#18131=CYLINDRICAL_SURFACE ( 'NONE', #15368, 0.9999999999999991118 ) ;
#18161=CARTESIAN_POINT ( 'NONE',  ( 2.449293598294706513E-15, -20.00000000000000000, 9.000000000000000000 ) ) ;
#18164=EDGE_CURVE ( 'NONE', #17065, #8420, #5891, .T. ) ;
#18167=CARTESIAN_POINT ( 'NONE',  ( -19.89043790736547379, -17.90943073464699609, 9.000000000000000000 ) ) ;
#18176=DIRECTION ( 'NONE',  ( 0.000000000000000000, 0.000000000000000000, -1.000000000000000000 ) ) ;
#18177=DIRECTION ( 'NONE',  ( 0.000000000000000000, 0.000000000000000000, 1.000000000000000000 ) ) ;
#18186=DIRECTION ( 'NONE',  ( 0.000000000000000000, -0.000000000000000000, -1.000000000000000000 ) ) ;
#18202=DIRECTION ( 'NONE',  ( -1.000000000000000000, 0.000000000000000000, 0.000000000000000000 ) ) ;
#18213=ORIENTED_EDGE ( 'NONE', *, *, #14897, .F. ) ;
#18214=EDGE_CURVE ( 'NONE', #4891, #4202, #1581, .T. ) ;
#18226=CIRCLE ( 'NONE', #10355, 0.9999999999999982236 ) ;
#18235=VERTEX_POINT ( 'NONE', #11963 ) ;
#18238=CIRCLE ( 'NONE', #9747, 1.000000000000000000 ) ;
#18240=( GEOMETRIC_REPRESENTATION_CONTEXT ( 3 ) GLOBAL_UNCERTAINTY_ASSIGNED_CONTEXT ( ( #2069 ) ) GLOBAL_UNIT_ASSIGNED_CONTEXT ( ( #15917, #12875, #11389 ) ) REPRESENTATION_CONTEXT ( 'NONE', 'WORKASPACE' ) );
#18243=CARTESIAN_POINT ( 'NONE',  ( 4.158233816355333623, -39.56295201467608535, -9.000000000000000000 ) ) ;
#18250=CARTESIAN_POINT ( 'NONE',  ( -19.30627432446647163, -14.77814480204146363, 0.000000000000000000 ) ) ;
#18271=DIRECTION ( 'NONE',  ( -1.000000000000000000, 0.000000000000000000, 0.000000000000000000 ) ) ;
#18276=DIRECTION ( 'NONE',  ( 0.000000000000000000, 0.000000000000000000, 1.000000000000000000 ) ) ;
#18292=CARTESIAN_POINT ( 'NONE',  ( -7.211304515372564339, -38.65468003441944234, 0.000000000000000000 ) ) ;
#18299=ADVANCED_FACE ( 'NONE', ( #300 ), #1771, .T. ) ;
#18312=EDGE_LOOP ( 'NONE', ( #4434, #9847, #18920, #14558 ) ) ;
#18314=VECTOR ( 'NONE', #18176, 1000.000000000000000 ) ;
#18334=DIRECTION ( 'NONE',  ( -0.000000000000000000, -0.000000000000000000, -1.000000000000000000 ) ) ;
#18344=AXIS2_PLACEMENT_3D ( 'NONE', #2836, #7137, #11932 ) ;
#18347=EDGE_CURVE ( 'NONE', #660, #18235, #313, .T. ) ;
#18348=CARTESIAN_POINT ( 'NONE',  ( 8.134732861516145164, -38.27090915285195649, -9.000000000000000000 ) ) ;
#18356=ORIENTED_EDGE ( 'NONE', *, *, #7232, .F. ) ;
#18363=CARTESIAN_POINT ( 'NONE',  ( -8.134732861516020819, -1.729090847147989773, -9.000000000000000000 ) ) ;
#18374=VECTOR ( 'NONE', #2734, 1000.000000000000000 ) ;
#18383=AXIS2_PLACEMENT_3D ( 'NONE', #17998, #7395, #9053 ) ;
#18391=EDGE_CURVE ( 'NONE', #6328, #16520, #6576, .T. ) ;
#18392=CARTESIAN_POINT ( 'NONE',  ( 2.449293598294706513E-15, -20.00000000000000000, 9.000000000000000000 ) ) ;
#18396=EDGE_CURVE ( 'NONE', #1857, #3727, #17871, .T. ) ;
#18398=ORIENTED_EDGE ( 'NONE', *, *, #3289, .F. ) ;
#18400=AXIS2_PLACEMENT_3D ( 'NONE', #9870, #15865, #2447 ) ;
#18401=ORIENTED_EDGE ( 'NONE', *, *, #10396, .T. ) ;
#18402=EDGE_CURVE ( 'NONE', #6795, #1052, #17424, .T. ) ;
#18404=ORIENTED_EDGE ( 'NONE', *, *, #1991, .F. ) ;
#18412=ADVANCED_FACE ( 'NONE', ( #1139 ), #15754, .F. ) ;
#18425=CARTESIAN_POINT ( 'NONE',  ( -3.175194142252082852, -39.74634503291706267, 0.000000000000000000 ) ) ;
#18443=( GEOMETRIC_REPRESENTATION_CONTEXT ( 3 ) GLOBAL_UNCERTAINTY_ASSIGNED_CONTEXT ( ( #5986 ) ) GLOBAL_UNIT_ASSIGNED_CONTEXT ( ( #5282, #3825, #978 ) ) REPRESENTATION_CONTEXT ( 'NONE', 'WORKASPACE' ) );
#18444=VERTEX_POINT ( 'NONE', #14263 ) ;
#18450=CARTESIAN_POINT ( 'NONE',  ( 19.97007065299861139, -18.90625500492856759, -9.000000000000000000 ) ) ;
#18456=EDGE_CURVE ( 'NONE', #11695, #9447, #2198, .T. ) ;
#18457=CARTESIAN_POINT ( 'NONE',  ( -3.158233816355195955, -0.4370479853238878887, -9.000000000000000000 ) ) ;
#18465=AXIS2_PLACEMENT_3D ( 'NONE', #16219, #6024, #7089 ) ;
#18468=CARTESIAN_POINT ( 'NONE',  ( -18.89043790736545603, -22.09056926535314602, 9.000000000000000000 ) ) ;
#18475=AXIS2_PLACEMENT_3D ( 'NONE', #2161, #14098, #6459 ) ;
#18484=CARTESIAN_POINT ( 'NONE',  ( 2.449293598294706513E-15, -20.00000000000000000, 9.000000000000000000 ) ) ;
#18486=CARTESIAN_POINT ( 'NONE',  ( -17.32050807568879236, -10.00000000000004263, 9.000000000000000000 ) ) ;
#18493=AXIS2_PLACEMENT_3D ( 'NONE', #7318, #15153, #159 ) ;
#18497=EDGE_CURVE ( 'NONE', #12683, #15949, #847, .T. ) ;
#18499=AXIS2_PLACEMENT_3D ( 'NONE', #19002, #16049, #6919 ) ;
#18520=DIRECTION ( 'NONE',  ( 4.082155997157843695E-16, -1.000000000000000000, 0.000000000000000000 ) ) ;
#18532=VERTEX_POINT ( 'NONE', #6129 ) ;
#18541=ADVANCED_FACE ( 'NONE', ( #61 ), #7501, .T. ) ;
#18547=AXIS2_PLACEMENT_3D ( 'NONE', #9260, #12111, #4683 ) ;
#18550=VECTOR ( 'NONE', #19225, 1000.000000000000000 ) ;
#18555=DIRECTION ( 'NONE',  ( 1.000000000000000000, 0.000000000000000000, 0.000000000000000000 ) ) ;
#18559=VERTEX_POINT ( 'NONE', #9060 ) ;
#18560=DIRECTION ( 'NONE',  ( -0.9135454576426043083, 0.4067366430757925477, 0.000000000000000000 ) ) ;
#18570=AXIS2_PLACEMENT_3D ( 'NONE', #7496, #13374, #2998 ) ;
#18580=DIRECTION ( 'NONE',  ( -0.000000000000000000, -0.000000000000000000, 1.000000000000000000 ) ) ;
#18606=DIRECTION ( 'NONE',  ( 0.000000000000000000, -0.000000000000000000, 1.000000000000000000 ) ) ;
#18628=LINE ( 'NONE', #3425, #4744 ) ;
#18640=CARTESIAN_POINT ( 'NONE',  ( -14.86289650954781649, -33.38261212717723936, -9.000000000000000000 ) ) ;
#18641=ADVANCED_FACE ( 'NONE', ( #2811 ), #4370, .F. ) ;
#18673=DIRECTION ( 'NONE',  ( 0.000000000000000000, 0.000000000000000000, -1.000000000000000000 ) ) ;
#18676=FACE_OUTER_BOUND ( 'NONE', #17089, .T. ) ;
#18683=AXIS2_PLACEMENT_3D ( 'NONE', #18053, #16387, #14898 ) ;
#18686=FACE_OUTER_BOUND ( 'NONE', #16547, .T. ) ;
#18687=ORIENTED_EDGE ( 'NONE', *, *, #1733, .F. ) ;
#18695=CARTESIAN_POINT ( 'NONE',  ( -3.175194142252069973, -39.74634503291706267, -9.000000000000000000 ) ) ;
#18711=ORIENTED_EDGE ( 'NONE', *, *, #116, .T. ) ;
#18715=DIRECTION ( 'NONE',  ( -0.000000000000000000, -0.000000000000000000, -1.000000000000000000 ) ) ;
#18719=AXIS2_PLACEMENT_3D ( 'NONE', #12866, #14430, #13057 ) ;
#18722=EDGE_LOOP ( 'NONE', ( #15392, #12112, #16798, #14191 ) ) ;
#18727=CARTESIAN_POINT ( 'NONE',  ( 2.449293598294706513E-15, -20.00000000000000000, 9.000000000000000000 ) ) ;
#18731=ORIENTED_EDGE ( 'NONE', *, *, #16722, .T. ) ;
#18733=VECTOR ( 'NONE', #5636, 1000.000000000000000 ) ;
#18737=CYLINDRICAL_SURFACE ( 'NONE', #19132, 1.000000000000000888 ) ;
#18738=ORIENTED_EDGE ( 'NONE', *, *, #281, .T. ) ;
#18752=EDGE_CURVE ( 'NONE', #16440, #10629, #13471, .T. ) ;
#18762=CARTESIAN_POINT ( 'NONE',  ( 2.449293598294706513E-15, -20.00000000000000000, 9.000000000000000000 ) ) ;
#18771=AXIS2_PLACEMENT_3D ( 'NONE', #17042, #462, #12415 ) ;
#18791=DIRECTION ( 'NONE',  ( -0.000000000000000000, -0.000000000000000000, 1.000000000000000000 ) ) ;
#18795=CARTESIAN_POINT ( 'NONE',  ( -7.211304515372564339, -38.65468003441944234, 9.000000000000000000 ) ) ;
#18798=CYLINDRICAL_SURFACE ( 'NONE', #14201, 1.000000000000000888 ) ;
#18803=AXIS2_PLACEMENT_3D ( 'NONE', #17770, #13340, #4231 ) ;
#18806=CARTESIAN_POINT ( 'NONE',  ( -19.02113032590308705, -13.81966011250110249, -9.000000000000000000 ) ) ;
#18808=ADVANCED_FACE ( 'NONE', ( #8167 ), #14527, .F. ) ;
#18823=AXIS2_PLACEMENT_3D ( 'NONE', #5467, #11350, #8407 ) ;
#18844=VERTEX_POINT ( 'NONE', #11394 ) ;
#18853=AXIS2_PLACEMENT_3D ( 'NONE', #12963, #13163, #5720 ) ;
#18855=DIRECTION ( 'NONE',  ( 0.9781476007338055778, 0.2079116908177597867, 0.000000000000000000 ) ) ;
#18858=DIRECTION ( 'NONE',  ( 1.000000000000000000, 0.000000000000000000, 0.000000000000000000 ) ) ;
#18866=CARTESIAN_POINT ( 'NONE',  ( -19.76107906696388739, -23.08216711247161967, -9.000000000000000000 ) ) ;
#18871=CARTESIAN_POINT ( 'NONE',  ( 18.68843350152485172, -12.87662627267922666, -9.000000000000000000 ) ) ;
#18885=PLANE ( 'NONE',  #9349 ) ;
#18888=EDGE_CURVE ( 'NONE', #12892, #11553, #632, .T. ) ;
#18901=CARTESIAN_POINT ( 'NONE',  ( 12.54977455159103705, -4.427487078051979275, 9.000000000000000000 ) ) ;
#18917=CYLINDRICAL_SURFACE ( 'NONE', #19311, 1.000000000000000888 ) ;
#18920=ORIENTED_EDGE ( 'NONE', *, *, #1026, .T. ) ;
#18925=DIRECTION ( 'NONE',  ( 0.5000000000000108802, -0.8660254037844323793, 0.000000000000000000 ) ) ;
#18928=CIRCLE ( 'NONE', #16415, 20.00000000000000000 ) ;
#18930=ORIENTED_EDGE ( 'NONE', *, *, #13338, .T. ) ;
#18931=VERTEX_POINT ( 'NONE', #4343 ) ;
#18937=ORIENTED_EDGE ( 'NONE', *, *, #10706, .T. ) ;
#18954=CARTESIAN_POINT ( 'NONE',  ( 5.130877905917419213, -39.33065161639846252, 9.000000000000000000 ) ) ;
#18957=EDGE_LOOP ( 'NONE', ( #15111, #1946, #9718, #17500 ) ) ;
#18958=CIRCLE ( 'NONE', #7038, 1.000000000000000222 ) ;
#18959=DIRECTION ( 'NONE',  ( 0.000000000000000000, 0.000000000000000000, 1.000000000000000000 ) ) ;
#18963=DIRECTION ( 'NONE',  ( -1.000000000000000000, 0.000000000000000000, 0.000000000000000000 ) ) ;
#18974=FACE_OUTER_BOUND ( 'NONE', #8044, .T. ) ;
#18980=ORIENTED_EDGE ( 'NONE', *, *, #4020, .T. ) ;
#18991=AXIS2_PLACEMENT_3D ( 'NONE', #18040, #1461, #15178 ) ;
#19000=AXIS2_PLACEMENT_3D ( 'NONE', #15382, #15189, #1962 ) ;
#19001=DIRECTION ( 'NONE',  ( 0.000000000000000000, 0.000000000000000000, 1.000000000000000000 ) ) ;
#19002=CARTESIAN_POINT ( 'NONE',  ( 2.449293598294706513E-15, -20.00000000000000000, 9.000000000000000000 ) ) ;
#19006=CARTESIAN_POINT ( 'NONE',  ( -19.76107906696391225, -16.91783288752853665, 0.000000000000000000 ) ) ;
#19012=VERTEX_POINT ( 'NONE', #8751 ) ;
#19018=ORIENTED_EDGE ( 'NONE', *, *, #5411, .F. ) ;
#19026=DIRECTION ( 'NONE',  ( 0.000000000000000000, 0.000000000000000000, 1.000000000000000000 ) ) ;
#19030=EDGE_LOOP ( 'NONE', ( #5165, #16462, #17347, #19059 ) ) ;
#19034=CARTESIAN_POINT ( 'NONE',  ( 19.76107906696387673, -16.91783288752826664, 0.000000000000000000 ) ) ;
#19040=CARTESIAN_POINT ( 'NONE',  ( 8.134732861515777458, -1.729090847147875198, -9.000000000000000000 ) ) ;
#19058=CIRCLE ( 'NONE', #10262, 1.000000000000000444 ) ;
#19059=ORIENTED_EDGE ( 'NONE', *, *, #5807, .F. ) ;
#19060=CARTESIAN_POINT ( 'NONE',  ( 2.449293598294706513E-15, -20.00000000000000000, 9.000000000000000000 ) ) ;
#19073=DIRECTION ( 'NONE',  ( -0.3090169943749382919, -0.9510565162951566398, 0.000000000000000000 ) ) ;
#19075=CIRCLE ( 'NONE', #10890, 20.00000000000000000 ) ;
#19085=DIRECTION ( 'NONE',  ( 1.000000000000000000, 0.000000000000000000, 0.000000000000000000 ) ) ;
#19092=FACE_OUTER_BOUND ( 'NONE', #15444, .T. ) ;
#19111=VERTEX_POINT ( 'NONE', #10504 ) ;
#19128=ORIENTED_EDGE ( 'NONE', *, *, #15518, .T. ) ;
#19132=AXIS2_PLACEMENT_3D ( 'NONE', #8027, #5286, #14003 ) ;
#19135=VECTOR ( 'NONE', #13236, 1000.000000000000000 ) ;
#19138=DIRECTION ( 'NONE',  ( 0.000000000000000000, 0.000000000000000000, 1.000000000000000000 ) ) ;
#19140=AXIS2_PLACEMENT_3D ( 'NONE', #10143, #17331, #3890 ) ;
#19143=DIRECTION ( 'NONE',  ( -0.000000000000000000, -0.000000000000000000, 1.000000000000000000 ) ) ;
#19146=CIRCLE ( 'NONE', #16949, 0.9999999999999982236 ) ;
#19148=DIRECTION ( 'NONE',  ( -0.000000000000000000, 0.000000000000000000, -1.000000000000000000 ) ) ;
#19159=EDGE_LOOP ( 'NONE', ( #13078, #4458, #10486, #8855 ) ) ;
#19160=DIRECTION ( 'NONE',  ( 0.000000000000000000, 0.000000000000000000, 1.000000000000000000 ) ) ;
#19164=CIRCLE ( 'NONE', #10003, 0.9999999999999995559 ) ;
#19165=DIRECTION ( 'NONE',  ( 0.000000000000000000, 0.000000000000000000, 1.000000000000000000 ) ) ;
#19176=DIRECTION ( 'NONE',  ( 0.000000000000000000, 0.000000000000000000, 1.000000000000000000 ) ) ;
#19179=EDGE_CURVE ( 'NONE', #12796, #11041, #3361, .T. ) ;
#19181=AXIS2_PLACEMENT_3D ( 'NONE', #12307, #4867, #5630 ) ;
#19188=ORIENTED_EDGE ( 'NONE', *, *, #3423, .T. ) ;
#19191=DIRECTION ( 'NONE',  ( -0.000000000000000000, -0.000000000000000000, -1.000000000000000000 ) ) ;
#19196=LINE ( 'NONE', #14459, #2656 ) ;
#19197=ADVANCED_FACE ( 'NONE', ( #9323 ), #3265, .F. ) ;
#19215=DIRECTION ( 'NONE',  ( -0.000000000000000000, -0.000000000000000000, -1.000000000000000000 ) ) ;
#19217=EDGE_LOOP ( 'NONE', ( #13194, #7609, #6021, #1611 ) ) ;
#19225=DIRECTION ( 'NONE',  ( 0.000000000000000000, -0.000000000000000000, -1.000000000000000000 ) ) ;
#19226=CARTESIAN_POINT ( 'NONE',  ( 19.02113032590300890, -13.81966011250085025, -9.000000000000000000 ) ) ;
#19242=EDGE_CURVE ( 'NONE', #10464, #15949, #10031, .T. ) ;
#19244=DIRECTION ( 'NONE',  ( 0.000000000000000000, 0.000000000000000000, 1.000000000000000000 ) ) ;
#19257=ORIENTED_EDGE ( 'NONE', *, *, #13276, .T. ) ;
#19261=AXIS2_PLACEMENT_3D ( 'NONE', #1493, #15116, #16404 ) ;
#19265=CYLINDRICAL_SURFACE ( 'NONE', #12130, 5.000000000000000888 ) ;
#19267=CARTESIAN_POINT ( 'NONE',  ( 11.75570504584960041, -36.18033988749885310, -9.000000000000000000 ) ) ;
#19280=CARTESIAN_POINT ( 'NONE',  ( 12.54977455159135502, -35.57251292194776227, 9.000000000000000000 ) ) ;
#19289=ORIENTED_EDGE ( 'NONE', *, *, #10698, .F. ) ;
#19292=DIRECTION ( 'NONE',  ( 0.000000000000000000, 0.000000000000000000, 1.000000000000000000 ) ) ;
#19295=EDGE_CURVE ( 'NONE', #4327, #508, #12223, .T. ) ;
#19305=ORIENTED_EDGE ( 'NONE', *, *, #10698, .T. ) ;
#19308=CARTESIAN_POINT ( 'NONE',  ( -19.97007065299860784, -21.09374499507130452, 9.000000000000000000 ) ) ;
#19309=ORIENTED_EDGE ( 'NONE', *, *, #10206, .T. ) ;
#19311=AXIS2_PLACEMENT_3D ( 'NONE', #1248, #5458, #5367 ) ;
#19314=ORIENTED_EDGE ( 'NONE', *, *, #16042, .F. ) ;
#19354=VECTOR ( 'NONE', #2051, 1000.000000000000000 ) ;
#19360=CIRCLE ( 'NONE', #2747, 1.000000000000000666 ) ;
#19367=CYLINDRICAL_SURFACE ( 'NONE', #14217, 1.000000000000000888 ) ;
#19393=DIRECTION ( 'NONE',  ( 1.000000000000000000, 0.000000000000000000, 0.000000000000000000 ) ) ;
#19396=EDGE_CURVE ( 'NONE', #13178, #12683, #16323, .T. ) ;
#19404=ORIENTED_EDGE ( 'NONE', *, *, #3457, .F. ) ;
#19409=DIRECTION ( 'NONE',  ( -0.000000000000000000, -0.000000000000000000, 1.000000000000000000 ) ) ;
#19410=CARTESIAN_POINT ( 'NONE',  ( 19.30627432446641123, -14.77814480204120784, -9.000000000000000000 ) ) ;
#19448=COLOUR_RGB('Light Blue',0.38,0.62,0.78);
#19449=FILL_AREA_STYLE_COLOUR('',#19448);
#19450=FILL_AREA_STYLE('',(#19449));
#19451=SURFACE_STYLE_FILL_AREA(#19450);
#19452=SURFACE_SIDE_STYLE('',(#19451));
#19453=SURFACE_STYLE_USAGE(.BOTH.,#19452);
#19454=PRESENTATION_STYLE_ASSIGNMENT((#19453));
ENDSEC;
END-ISO-10303-21;
